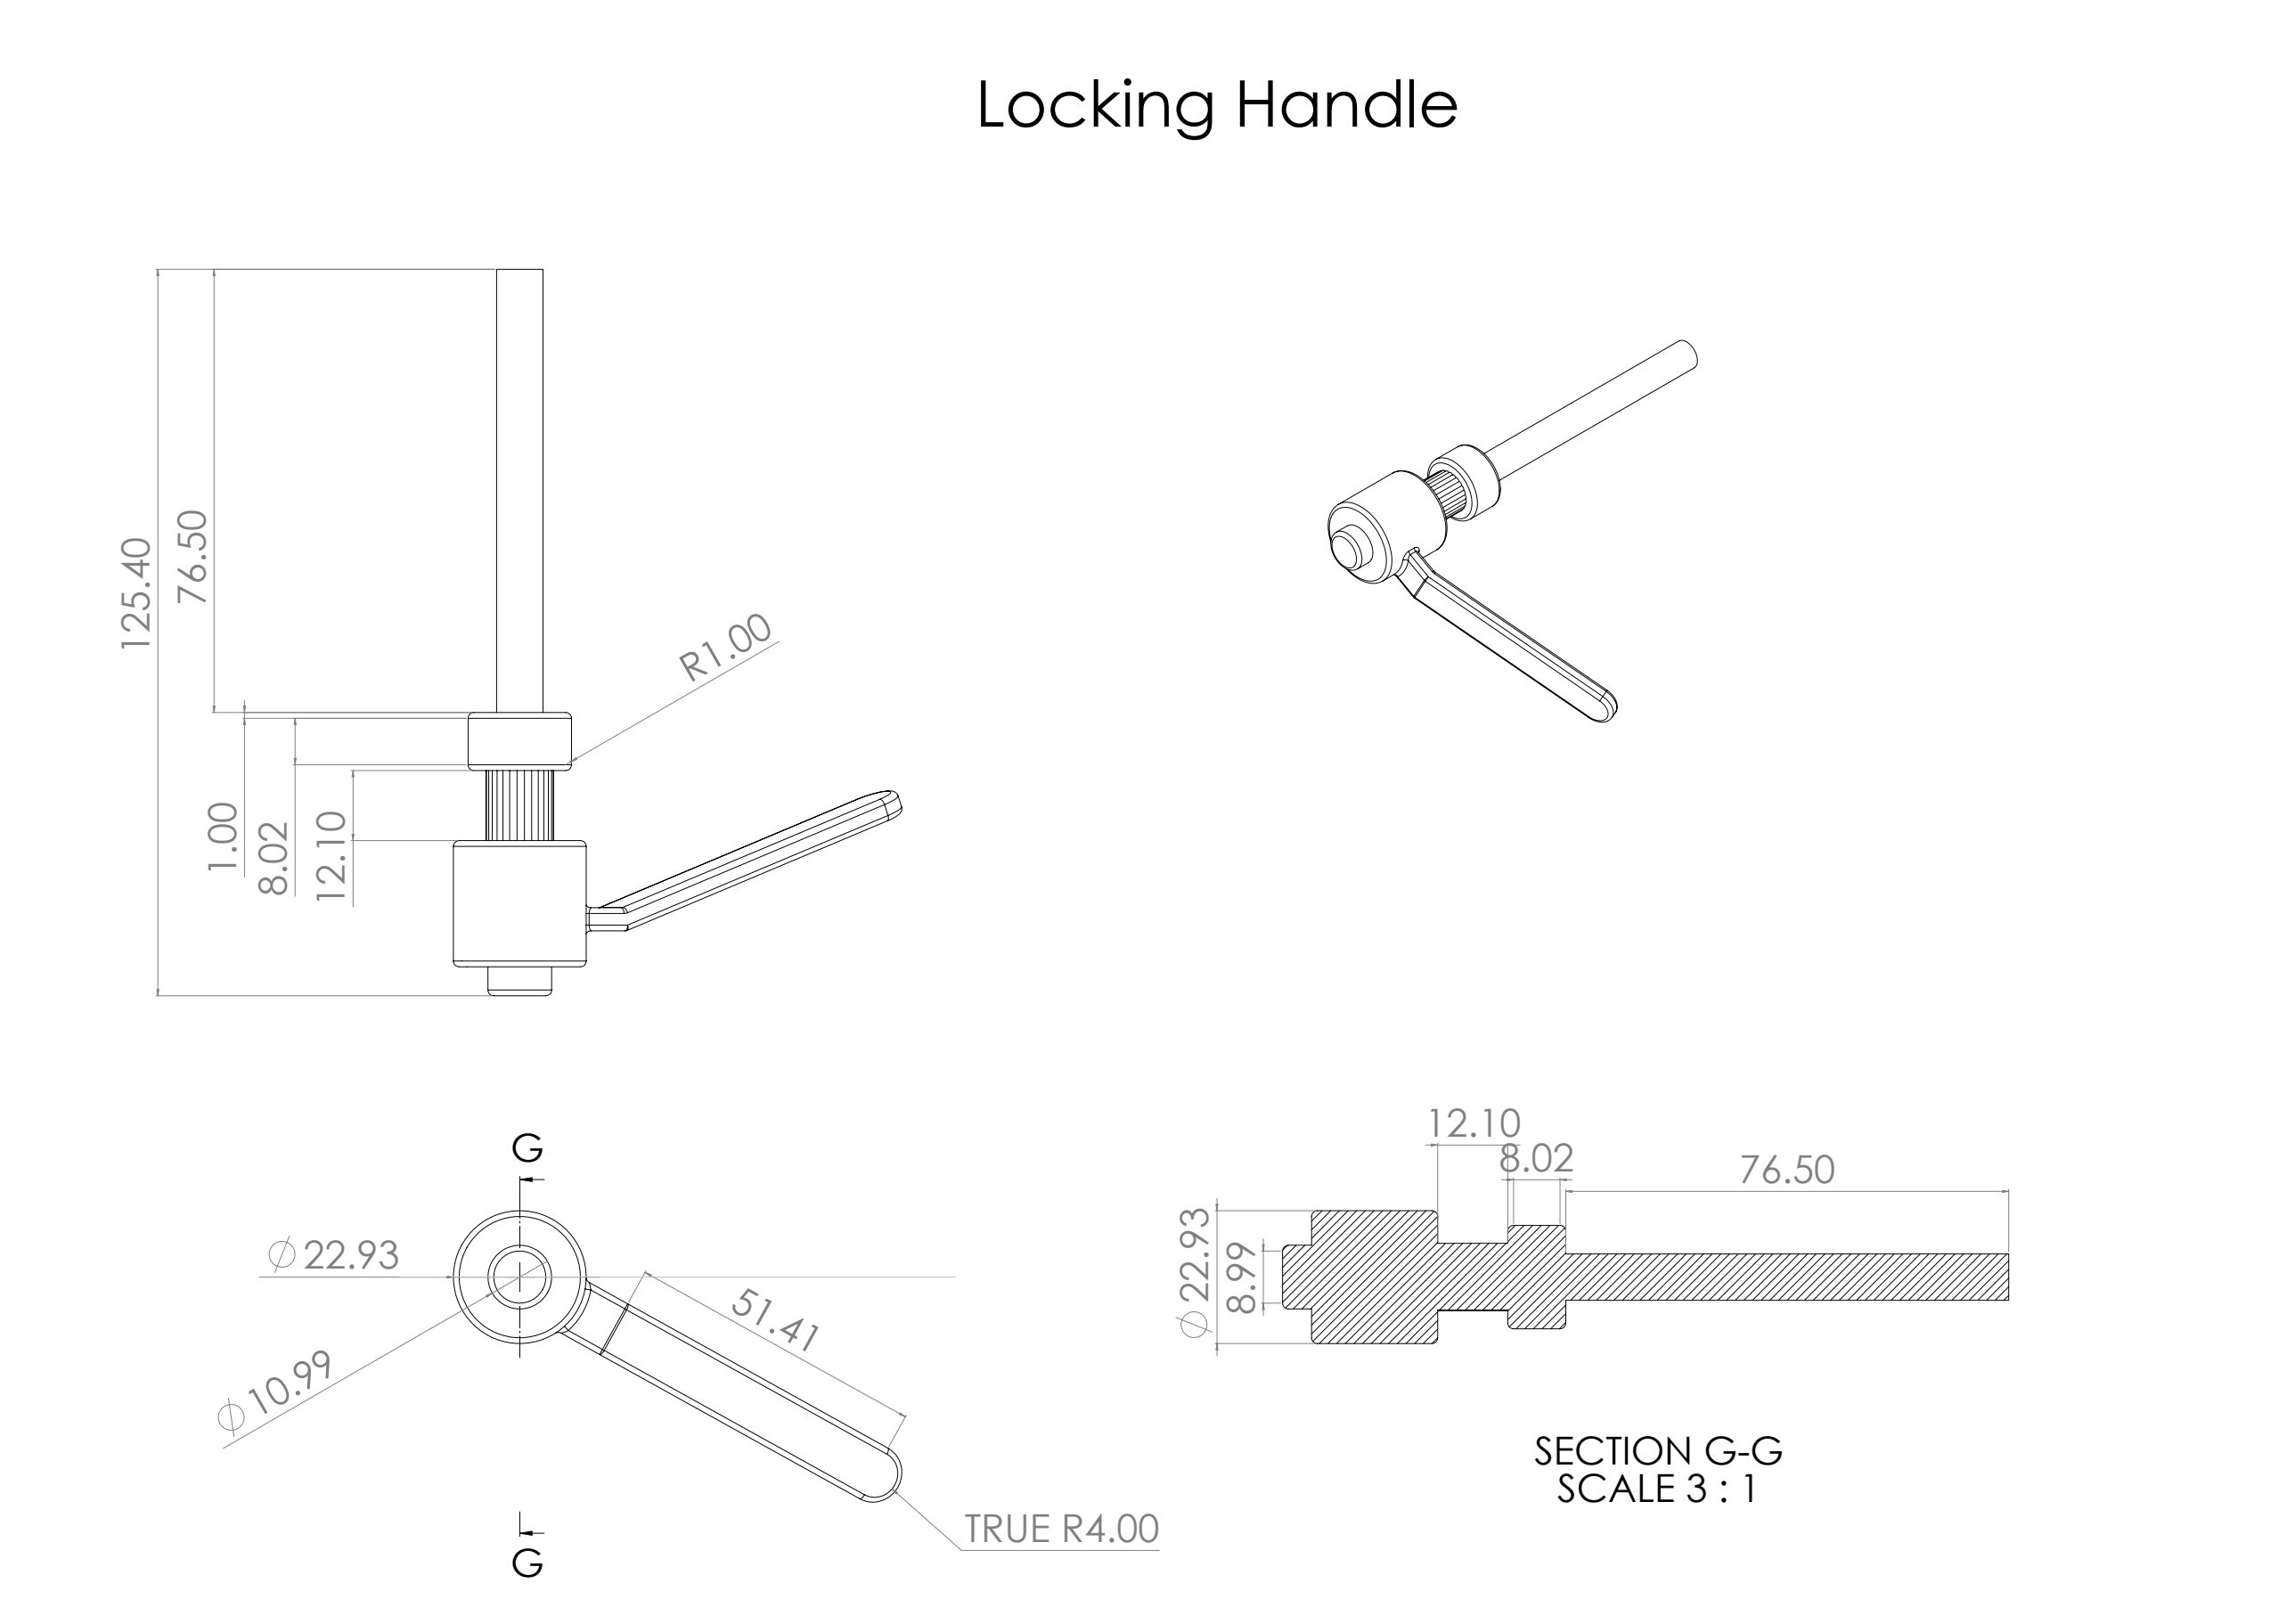
ISO-10303-21;
HEADER;
FILE_DESCRIPTION (('STEP AP214'),
    '1' );
FILE_NAME ('Locking Handle.step',
    '2026-10-24T21:31:31',
    ( '' ),
    ( '' ),
    'SwSTEP 2.0',
    'SolidWorks 2025',
    '' );
FILE_SCHEMA (( 'AUTOMOTIVE_DESIGN' ));
ENDSEC;

DATA;
#2=CARTESIAN_POINT ( 'NONE',  ( 58.00000000000000711, -2.249290599286309256, 86.40005259842790508 ) ) ;
#3=CARTESIAN_POINT ( 'NONE',  ( 58.00000000000000711, -2.249290599286309256, 86.40005259842790508 ) ) ;
#7=CARTESIAN_POINT ( 'NONE',  ( 64.16497654487091040, -11.91588057969686965, 72.65167857827074727 ) ) ;
#22=DIRECTION ( 'NONE',  ( 0.000000000000000000, 0.000000000000000000, -1.000000000000000000 ) ) ;
#23=FACE_OUTER_BOUND ( 'NONE', #14250, .T. ) ;
#26=DIRECTION ( 'NONE',  ( -0.8746197071345572782, 0.4848096202550659650, 1.387778780781444256E-14 ) ) ;
#27=ADVANCED_FACE ( 'NONE', ( #435 ), #1875, .T. ) ;
#30=EDGE_CURVE ( 'NONE', #1762, #13149, #4870, .T. ) ;
#35=CIRCLE ( 'NONE', #11822, 8.924024642120691908 ) ;
#39=DIRECTION ( 'NONE',  ( -0.3020115420618247892, 0.1674077314120183957, -0.9384901064608620613 ) ) ;
#40=CARTESIAN_POINT ( 'NONE',  ( 62.00000000000001421, -2.249290599286311032, -49.31370849898490150 ) ) ;
#43=CARTESIAN_POINT ( 'NONE',  ( 116.3214526938479025, -39.15081599364015119, 53.46824312087640863 ) ) ;
#44=AXIS2_PLACEMENT_3D ( 'NONE', #5649, #10264, #10339 ) ;
#59=VERTEX_POINT ( 'NONE', #10047 ) ;
#61=CARTESIAN_POINT ( 'NONE',  ( 65.61438479068812057, -11.78561916032472823, 75.96106737140233633 ) ) ;
#74=EDGE_CURVE ( 'NONE', #5063, #10163, #11263, .T. ) ;
#76=ORIENTED_EDGE ( 'NONE', *, *, #9899, .T. ) ;
#79=ORIENTED_EDGE ( 'NONE', *, *, #10646, .T. ) ;
#84=DIRECTION ( 'NONE',  ( -0.000000000000000000, 0.000000000000000000, -1.000000000000000000 ) ) ;
#85=ORIENTED_EDGE ( 'NONE', *, *, #4287, .T. ) ;
#100=DIRECTION ( 'NONE',  ( -0.8746197071345569451, 0.4848096202550666312, 0.000000000000000000 ) ) ;
#117=VERTEX_POINT ( 'NONE', #8210 ) ;
#121=CARTESIAN_POINT ( 'NONE',  ( 54.21883389619742388, -5.612936290787406968, 62.84860122826521689 ) ) ;
#124=CARTESIAN_POINT ( 'NONE',  ( 69.30309607900824176, -4.171217477998490075, 76.23845400177138742 ) ) ;
#128=FACE_BOUND ( 'NONE', #8065, .T. ) ;
#136=CARTESIAN_POINT ( 'NONE',  ( 64.12616288941416087, -11.93994285747185913, 75.47114622899779590 ) ) ;
#137=CARTESIAN_POINT ( 'NONE',  ( 65.80512781895316721, -6.575743597179694255, 39.50000000000012790 ) ) ;
#140=ADVANCED_FACE ( 'NONE', ( #6968 ), #10511, .T. ) ;
#141=CARTESIAN_POINT ( 'NONE',  ( 59.31076468612580754, 2.638779099491020297, 60.61639468829817190 ) ) ;
#142=CARTESIAN_POINT ( 'NONE',  ( 67.15257324181105503, -7.322644791425994448, 61.61639468829817190 ) ) ;
#144=CARTESIAN_POINT ( 'NONE',  ( 65.51787304867481510, -10.90583193546819274, 77.18393887567587797 ) ) ;
#147=ORIENTED_EDGE ( 'NONE', *, *, #2886, .F. ) ;
#149=AXIS2_PLACEMENT_3D ( 'NONE', #12314, #13325, #4001 ) ;
#150=ORIENTED_EDGE ( 'NONE', *, *, #12236, .T. ) ;
#152=CARTESIAN_POINT ( 'NONE',  ( 65.93900958890544928, -0.9331851346922672708, 76.19766410831374515 ) ) ;
#153=VERTEX_POINT ( 'NONE', #5752 ) ;
#156=EDGE_LOOP ( 'NONE', ( #7728, #5694, #9406, #597 ) ) ;
#159=TOROIDAL_SURFACE ( 'NONE', #9985, 10.46463184759104870, 1.000000000000000000 ) ;
#178=LINE ( 'NONE', #7254, #6578 ) ;
#179=FACE_OUTER_BOUND ( 'NONE', #4257, .T. ) ;
#185=CARTESIAN_POINT ( 'NONE',  ( 121.8459904851758893, -37.63970102501964021, 53.02550872668530246 ) ) ;
#192=CIRCLE ( 'NONE', #14918, 0.7892041907098250597 ) ;
#195=CARTESIAN_POINT ( 'NONE',  ( 65.61529858912808777, -10.82031860958136704, 71.19766410831375936 ) ) ;
#196=EDGE_CURVE ( 'NONE', #211, #4051, #4578, .T. ) ;
#199=AXIS2_PLACEMENT_3D ( 'NONE', #2893, #5282, #2974 ) ;
#207=EDGE_CURVE ( 'NONE', #5032, #7204, #4344, .T. ) ;
#211=VERTEX_POINT ( 'NONE', #3190 ) ;
#213=DIRECTION ( 'NONE',  ( 0.000000000000000000, 0.000000000000000000, -1.000000000000000000 ) ) ;
#225=ORIENTED_EDGE ( 'NONE', *, *, #12393, .F. ) ;
#230=EDGE_CURVE ( 'NONE', #13103, #13525, #1896, .T. ) ;
#232=DIRECTION ( 'NONE',  ( 0.8746197071345569451, -0.4848096202550666312, 0.000000000000000000 ) ) ;
#233=CARTESIAN_POINT ( 'NONE',  ( 63.00747169918385993, -1.516790343742004055, 62.84860122826521689 ) ) ;
#238=VECTOR ( 'NONE', #7025, 1000.000000000000000 ) ;
#242=EDGE_CURVE ( 'NONE', #604, #9712, #875, .T. ) ;
#243=ORIENTED_EDGE ( 'NONE', *, *, #2367, .F. ) ;
#248=CARTESIAN_POINT ( 'NONE',  ( 53.45023817967523172, -5.433760736713491468, 48.51982618741349285 ) ) ;
#260=AXIS2_PLACEMENT_3D ( 'NONE', #10023, #5325, #2943 ) ;
#268=DIRECTION ( 'NONE',  ( -0.8746197071345569451, 0.4848096202550666312, 0.000000000000000000 ) ) ;
#271=CARTESIAN_POINT ( 'NONE',  ( 69.97972559857380759, -3.172990593254280789, 75.19766410831374515 ) ) ;
#277=ORIENTED_EDGE ( 'NONE', *, *, #11092, .F. ) ;
#279=ORIENTED_EDGE ( 'NONE', *, *, #8747, .F. ) ;
#281=ORIENTED_EDGE ( 'NONE', *, *, #7345, .T. ) ;
#283=CARTESIAN_POINT ( 'NONE',  ( 64.80908095809924419, -11.48972663575131392, 75.86800894915671734 ) ) ;
#285=DIRECTION ( 'NONE',  ( 0.8746197071345571672, -0.4848096202550661871, 0.000000000000000000 ) ) ;
#293=AXIS2_PLACEMENT_3D ( 'NONE', #12680, #6824, #7986 ) ;
#294=DIRECTION ( 'NONE',  ( -0.8746197071345569451, 0.4848096202550666312, 0.000000000000000000 ) ) ;
#297=TOROIDAL_SURFACE ( 'NONE', #10121, 4.496540510819672321, 1.000000000000000000 ) ;
#305=DIRECTION ( 'NONE',  ( 0.000000000000000000, 0.000000000000000000, 1.000000000000000000 ) ) ;
#306=DIRECTION ( 'NONE',  ( -0.000000000000000000, 0.000000000000000000, -1.000000000000000000 ) ) ;
#311=EDGE_CURVE ( 'NONE', #2576, #7654, #192, .T. ) ;
#317=ORIENTED_EDGE ( 'NONE', *, *, #10206, .F. ) ;
#318=VECTOR ( 'NONE', #6465, 1000.000000000000000 ) ;
#327=CYLINDRICAL_SURFACE ( 'NONE', #4362, 1.000000000000005329 ) ;
#334=DIRECTION ( 'NONE',  ( -0.8746197071345570562, 0.4848096202550662981, 0.000000000000000000 ) ) ;
#347=CARTESIAN_POINT ( 'NONE',  ( 69.46221311448613278, -2.886128737383383935, 75.38059407619712715 ) ) ;
#363=DIRECTION ( 'NONE',  ( 0.000000000000000000, 0.000000000000000000, 1.000000000000000000 ) ) ;
#364=EDGE_CURVE ( 'NONE', #14069, #12214, #5110, .T. ) ;
#367=DIRECTION ( 'NONE',  ( 0.000000000000000000, 0.000000000000000000, 1.000000000000000000 ) ) ;
#371=ORIENTED_EDGE ( 'NONE', *, *, #10491, .F. ) ;
#377=DIRECTION ( 'NONE',  ( 0.8746197071345570562, -0.4848096202550665756, 0.000000000000000000 ) ) ;
#381=CYLINDRICAL_SURFACE ( 'NONE', #9577, 11.46463184759105403 ) ;
#382=CARTESIAN_POINT ( 'NONE',  ( 50.19487218104683990, 2.077162398607073968, 82.40005259842790508 ) ) ;
#384=VERTEX_POINT ( 'NONE', #5940 ) ;
#393=DIRECTION ( 'NONE',  ( 1.000000000000000000, 0.000000000000000000, 0.000000000000000000 ) ) ;
#406=CARTESIAN_POINT ( 'NONE',  ( 57.51704887355756313, 3.283153786997079049, 60.61639468829817190 ) ) ;
#408=CYLINDRICAL_SURFACE ( 'NONE', #2891, 1.000000000000000888 ) ;
#412=AXIS2_PLACEMENT_3D ( 'NONE', #11507, #13599, #12438 ) ;
#416=CIRCLE ( 'NONE', #10992, 0.7892041907098262810 ) ;
#421=AXIS2_PLACEMENT_3D ( 'NONE', #800, #5514, #12747 ) ;
#423=VECTOR ( 'NONE', #6451, 1000.000000000000000 ) ;
#435=FACE_OUTER_BOUND ( 'NONE', #6645, .T. ) ;
#437=AXIS2_PLACEMENT_3D ( 'NONE', #3487, #8189, #5565 ) ;
#438=TOROIDAL_SURFACE ( 'NONE', #10274, 12.46463184759105047, 1.000000000000000000 ) ;
#453=LINE ( 'NONE', #3979, #12135 ) ;
#454=EDGE_LOOP ( 'NONE', ( #9894, #4373, #1618, #2467 ) ) ;
#464=DIRECTION ( 'NONE',  ( -0.8208219420614829565, 0.4549890321264266624, 0.3453061251629824246 ) ) ;
#471=EDGE_CURVE ( 'NONE', #12214, #14069, #7553, .T. ) ;
#477=AXIS2_PLACEMENT_3D ( 'NONE', #5498, #9026, #1017 ) ;
#482=DIRECTION ( 'NONE',  ( 1.000000000000000000, 0.000000000000000000, 0.000000000000000000 ) ) ;
#483=CARTESIAN_POINT ( 'NONE',  ( 62.00000000000001421, -2.249290599286311032, -38.00000000000012079 ) ) ;
#489=DIRECTION ( 'NONE',  ( -0.000000000000000000, 0.000000000000000000, -1.000000000000000000 ) ) ;
#496=ORIENTED_EDGE ( 'NONE', *, *, #8220, .F. ) ;
#506=EDGE_LOOP ( 'NONE', ( #7600, #11130, #5855, #5536 ) ) ;
#515=ORIENTED_EDGE ( 'NONE', *, *, #1099, .T. ) ;
#517=DIRECTION ( 'NONE',  ( 0.000000000000000000, 0.000000000000000000, -1.000000000000000000 ) ) ;
#518=EDGE_LOOP ( 'NONE', ( #85, #11509, #6587, #5049 ) ) ;
#524=FACE_BOUND ( 'NONE', #11436, .T. ) ;
#526=CARTESIAN_POINT ( 'NONE',  ( 68.02719294894561131, -7.807454411681060691, 82.40005259842790508 ) ) ;
#536=DIRECTION ( 'NONE',  ( -0.9249888031744268879, 0.3799943604870225089, 0.000000000000000000 ) ) ;
#539=CARTESIAN_POINT ( 'NONE',  ( 64.81656575362153205, -11.48379431191618671, 72.53457481663632223 ) ) ;
#547=CARTESIAN_POINT ( 'NONE',  ( 69.46454297106444642, -2.294433322023684774, 73.19766410831374515 ) ) ;
#553=AXIS2_PLACEMENT_3D ( 'NONE', #1342, #12818, #9352 ) ;
#556=VERTEX_POINT ( 'NONE', #13378 ) ;
#569=ORIENTED_EDGE ( 'NONE', *, *, #14553, .F. ) ;
#597=ORIENTED_EDGE ( 'NONE', *, *, #7672, .F. ) ;
#604=VERTEX_POINT ( 'NONE', #2615 ) ;
#607=DIRECTION ( 'NONE',  ( 0.000000000000000000, 0.000000000000000000, 1.000000000000000000 ) ) ;
#610=ADVANCED_FACE ( 'NONE', ( #2836 ), #381, .T. ) ;
#612=VERTEX_POINT ( 'NONE', #13245 ) ;
#614=CARTESIAN_POINT ( 'NONE',  ( 61.36510378087922390, 1.530577915148011225, 48.51982618741349285 ) ) ;
#629=DIRECTION ( 'NONE',  ( -0.000000000000000000, 0.000000000000000000, -1.000000000000000000 ) ) ;
#635=CARTESIAN_POINT ( 'NONE',  ( 58.00000000000000711, -2.249290599286309256, 61.61639468829817190 ) ) ;
#639=AXIS2_PLACEMENT_3D ( 'NONE', #12293, #305, #1535 ) ;
#644=AXIS2_PLACEMENT_3D ( 'NONE', #12063, #2755, #14382 ) ;
#650=ORIENTED_EDGE ( 'NONE', *, *, #10123, .F. ) ;
#653=EDGE_LOOP ( 'NONE', ( #6707, #7341, #9588, #14019 ) ) ;
#657=CARTESIAN_POINT ( 'NONE',  ( 64.11356537587559501, -11.94785244090458498, 73.19766410831374515 ) ) ;
#667=EDGE_CURVE ( 'NONE', #556, #7206, #3915, .T. ) ;
#679=CARTESIAN_POINT ( 'NONE',  ( 58.00000000000000711, -2.249290599286309256, 39.50000000000012790 ) ) ;
#682=CARTESIAN_POINT ( 'NONE',  ( 54.06723705530823310, -0.06932450177430288241, 87.40005259842790508 ) ) ;
#689=ORIENTED_EDGE ( 'NONE', *, *, #8732, .F. ) ;
#690=CARTESIAN_POINT ( 'NONE',  ( 69.97972559857382180, -3.172990593254281233, 73.19766410831374515 ) ) ;
#691=EDGE_CURVE ( 'NONE', #9315, #7200, #11147, .T. ) ;
#692=ADVANCED_FACE ( 'NONE', ( #8752 ), #5227, .T. ) ;
#695=CARTESIAN_POINT ( 'NONE',  ( 57.83740799265796539, -7.800393779465814248, 48.51982618741349285 ) ) ;
#697=CARTESIAN_POINT ( 'NONE',  ( 55.86211336638498182, 2.337731330496643167, 48.51982618741349285 ) ) ;
#702=DIRECTION ( 'NONE',  ( 0.8746197071345572782, -0.4848096202550659650, 0.000000000000000000 ) ) ;
#706=EDGE_CURVE ( 'NONE', #7249, #2361, #2636, .T. ) ;
#711=CARTESIAN_POINT ( 'NONE',  ( 55.09646579789918519, -6.394265699299607419, 48.51982618741349285 ) ) ;
#713=EDGE_LOOP ( 'NONE', ( #4880, #8165, #76, #1992, #12089, #15118, #2455, #11853, #2027, #8217 ) ) ;
#722=DIRECTION ( 'NONE',  ( -0.8746197071345572782, 0.4848096202550660205, 0.000000000000000000 ) ) ;
#724=CARTESIAN_POINT ( 'NONE',  ( 53.11142512232702018, -3.558169932106523881, 62.84860122826521689 ) ) ;
#739=ORIENTED_EDGE ( 'NONE', *, *, #13013, .T. ) ;
#740=EDGE_CURVE ( 'NONE', #6596, #11588, #12572, .T. ) ;
#742=CARTESIAN_POINT ( 'NONE',  ( 65.13162939602317181, -11.91918766459985157, 75.19766410831374515 ) ) ;
#756=CARTESIAN_POINT ( 'NONE',  ( 52.94134894379979528, -2.395505968190773327, 48.51982618741349285 ) ) ;
#758=AXIS2_PLACEMENT_3D ( 'NONE', #11179, #629, #8952 ) ;
#760=AXIS2_PLACEMENT_3D ( 'NONE', #3547, #3770, #5009 ) ;
#761=ORIENTED_EDGE ( 'NONE', *, *, #10485, .F. ) ;
#762=CARTESIAN_POINT ( 'NONE',  ( 69.99788034154117611, -3.225610097367463514, 75.50178636978743896 ) ) ;
#772=ORIENTED_EDGE ( 'NONE', *, *, #1941, .T. ) ;
#775=CARTESIAN_POINT ( 'NONE',  ( 52.25109540565180311, -2.012892184189035039, 62.84860122826521689 ) ) ;
#786=CYLINDRICAL_SURFACE ( 'NONE', #758, 0.7892041907098262810 ) ;
#787=ORIENTED_EDGE ( 'NONE', *, *, #10191, .T. ) ;
#795=CARTESIAN_POINT ( 'NONE',  ( 56.97758043373130477, 2.707118148285912795, 60.61639468829817190 ) ) ;
#796=DIRECTION ( 'NONE',  ( -0.000000000000000000, 0.000000000000000000, -1.000000000000000000 ) ) ;
#800=CARTESIAN_POINT ( 'NONE',  ( 62.80358567007132820, -3.842053655357405173, 60.61639468829817190 ) ) ;
#807=ORIENTED_EDGE ( 'NONE', *, *, #6638, .F. ) ;
#818=VECTOR ( 'NONE', #7680, 1000.000000000000000 ) ;
#819=FACE_OUTER_BOUND ( 'NONE', #7730, .T. ) ;
#833=CARTESIAN_POINT ( 'NONE',  ( 121.4079758241357609, -32.82348926221179397, 57.22220354671984666 ) ) ;
#846=CARTESIAN_POINT ( 'NONE',  ( 69.45807991563580686, -2.948854807202607731, 72.84297311730249191 ) ) ;
#852=ORIENTED_EDGE ( 'NONE', *, *, #5942, .T. ) ;
#854=( LENGTH_UNIT ( ) NAMED_UNIT ( * ) SI_UNIT ( .MILLI., .METRE. ) );
#858=ORIENTED_EDGE ( 'NONE', *, *, #14035, .T. ) ;
#860=DIRECTION ( 'NONE',  ( 0.9839406800755990945, -0.1784957649143745217, 0.000000000000000000 ) ) ;
#861=DIRECTION ( 'NONE',  ( -0.000000000000000000, 0.000000000000000000, -1.000000000000000000 ) ) ;
#865=ORIENTED_EDGE ( 'NONE', *, *, #8044, .F. ) ;
#873=CARTESIAN_POINT ( 'NONE',  ( 116.1386546156546444, -40.19284343218672007, 54.40673322733725570 ) ) ;
#875=LINE ( 'NONE', #15126, #9021 ) ;
#879=VERTEX_POINT ( 'NONE', #7688 ) ;
#885=CIRCLE ( 'NONE', #12695, 0.7892041907098275022 ) ;
#889=DIRECTION ( 'NONE',  ( 0.000000000000000000, 0.000000000000000000, 1.000000000000000000 ) ) ;
#899=FACE_OUTER_BOUND ( 'NONE', #4695, .T. ) ;
#900=ORIENTED_EDGE ( 'NONE', *, *, #4035, .F. ) ;
#909=AXIS2_PLACEMENT_3D ( 'NONE', #991, #9316, #8085 ) ;
#910=VECTOR ( 'NONE', #6269, 999.9999999999998863 ) ;
#924=CARTESIAN_POINT ( 'NONE',  ( 69.28051765693513175, -4.295678830383772961, 72.19766410831373094 ) ) ;
#931=VERTEX_POINT ( 'NONE', #8912 ) ;
#932=VECTOR ( 'NONE', #5247, 1000.000000000000000 ) ;
#940=ORIENTED_EDGE ( 'NONE', *, *, #12365, .F. ) ;
#943=VERTEX_POINT ( 'NONE', #12611 ) ;
#947=CARTESIAN_POINT ( 'NONE',  ( 60.05137561479872232, 2.911430354694811484, 48.51982618741349285 ) ) ;
#948=DIRECTION ( 'NONE',  ( -0.000000000000000000, 0.000000000000000000, -1.000000000000000000 ) ) ;
#959=ORIENTED_EDGE ( 'NONE', *, *, #13649, .F. ) ;
#978=DIRECTION ( 'NONE',  ( 0.3020115420618247892, -0.1674077314120183957, 0.9384901064608620613 ) ) ;
#983=DIRECTION ( 'NONE',  ( -0.4848096202550659650, -0.8746197071345572782, 0.000000000000000000 ) ) ;
#985=CARTESIAN_POINT ( 'NONE',  ( 54.00000000000000711, -2.249290599286310588, -49.31370849898490150 ) ) ;
#991=CARTESIAN_POINT ( 'NONE',  ( 58.00000000000000711, -2.249290599286311032, 38.50000000000012790 ) ) ;
#993=CARTESIAN_POINT ( 'NONE',  ( 69.41637355099324225, -3.305665566658139376, 76.92699484961572409 ) ) ;
#996=VERTEX_POINT ( 'NONE', #9154 ) ;
#999=AXIS2_PLACEMENT_3D ( 'NONE', #14231, #1449, #6157 ) ;
#1005=AXIS2_PLACEMENT_3D ( 'NONE', #15165, #10318, #12789 ) ;
#1010=EDGE_CURVE ( 'NONE', #879, #9712, #9431, .T. ) ;
#1016=CIRCLE ( 'NONE', #2502, 5.496540510819668768 ) ;
#1017=DIRECTION ( 'NONE',  ( 0.3020115420618323387, -0.1674077314120217264, 0.9384901064608589527 ) ) ;
#1020=ORIENTED_EDGE ( 'NONE', *, *, #14571, .F. ) ;
#1023=ORIENTED_EDGE ( 'NONE', *, *, #15171, .T. ) ;
#1024=DIRECTION ( 'NONE',  ( 0.1784957649143733838, 0.9839406800755994276, -0.000000000000000000 ) ) ;
#1033=DIRECTION ( 'NONE',  ( 0.8746197071345573892, -0.4848096202550657430, 0.000000000000000000 ) ) ;
#1040=EDGE_CURVE ( 'NONE', #12282, #6181, #9065, .T. ) ;
#1043=EDGE_CURVE ( 'NONE', #604, #5327, #4004, .T. ) ;
#1051=CARTESIAN_POINT ( 'NONE',  ( 68.02719294894561131, -7.807454411681058026, 81.40005259842790508 ) ) ;
#1052=DIRECTION ( 'NONE',  ( 0.000000000000000000, 0.000000000000000000, 1.000000000000000000 ) ) ;
#1056=ORIENTED_EDGE ( 'NONE', *, *, #10977, .T. ) ;
#1064=ORIENTED_EDGE ( 'NONE', *, *, #11189, .T. ) ;
#1065=DIRECTION ( 'NONE',  ( 0.000000000000000000, 0.000000000000000000, 1.000000000000000000 ) ) ;
#1067=CIRCLE ( 'NONE', #10913, 0.7892041907098261699 ) ;
#1068=EDGE_CURVE ( 'NONE', #2182, #12939, #10900, .T. ) ;
#1072=DIRECTION ( 'NONE',  ( -0.000000000000000000, 0.000000000000000000, -1.000000000000000000 ) ) ;
#1073=LINE ( 'NONE', #10467, #9643 ) ;
#1075=ORIENTED_EDGE ( 'NONE', *, *, #10722, .F. ) ;
#1077=CARTESIAN_POINT ( 'NONE',  ( 64.65840159946851884, -11.60091655178341696, 72.83455400280563197 ) ) ;
#1078=DIRECTION ( 'NONE',  ( 0.3020115420618247892, -0.1674077314120183957, 0.9384901064608620613 ) ) ;
#1087=DIRECTION ( 'NONE',  ( 0.000000000000000000, 0.000000000000000000, 1.000000000000000000 ) ) ;
#1088=CARTESIAN_POINT ( 'NONE',  ( 56.56161818778031858, -7.613266777470379942, 54.56811043785582882 ) ) ;
#1093=CARTESIAN_POINT ( 'NONE',  ( 54.30726695196912601, -6.397170215889376621, 60.61639468829817190 ) ) ;
#1094=CARTESIAN_POINT ( 'NONE',  ( 52.72873328492558187, -0.5014548242779776066, 54.56811043785582882 ) ) ;
#1099=EDGE_CURVE ( 'NONE', #3217, #9619, #12876, .T. ) ;
#1103=ORIENTED_EDGE ( 'NONE', *, *, #3765, .F. ) ;
#1118=FACE_OUTER_BOUND ( 'NONE', #3433, .T. ) ;
#1119=EDGE_CURVE ( 'NONE', #1157, #384, #4495, .T. ) ;
#1123=EDGE_CURVE ( 'NONE', #5327, #943, #11624, .T. ) ;
#1126=DIRECTION ( 'NONE',  ( 0.000000000000000000, 0.000000000000000000, 1.000000000000000000 ) ) ;
#1128=DIRECTION ( 'NONE',  ( 0.8746197071345569451, -0.4848096202550666312, 0.000000000000000000 ) ) ;
#1129=CYLINDRICAL_SURFACE ( 'NONE', #6973, 1.000000000000000444 ) ;
#1136=PLANE ( 'NONE',  #5436 ) ;
#1138=EDGE_LOOP ( 'NONE', ( #6793, #4822, #4988, #10304 ) ) ;
#1140=CARTESIAN_POINT ( 'NONE',  ( 54.17164678268019173, 2.103670757168142114, 60.61639468829817190 ) ) ;
#1147=AXIS2_PLACEMENT_3D ( 'NONE', #7440, #3671, #285 ) ;
#1154=DIRECTION ( 'NONE',  ( -0.8746197071345569451, 0.4848096202550666312, 0.000000000000000000 ) ) ;
#1157=VERTEX_POINT ( 'NONE', #6907 ) ;
#1168=ORIENTED_EDGE ( 'NONE', *, *, #11677, .T. ) ;
#1179=DIRECTION ( 'NONE',  ( -0.000000000000000000, 0.000000000000000000, -1.000000000000000000 ) ) ;
#1185=DIRECTION ( 'NONE',  ( -0.000000000000000000, -0.000000000000000000, -1.000000000000000000 ) ) ;
#1191=CARTESIAN_POINT ( 'NONE',  ( 71.15942379059755751, -15.26044865788734484, 71.19766410831374515 ) ) ;
#1192=DIRECTION ( 'NONE',  ( 0.000000000000000000, 0.000000000000000000, 1.000000000000000000 ) ) ;
#1207=CARTESIAN_POINT ( 'NONE',  ( 65.18141112804345028, -11.90723896596971798, 75.46703592544538708 ) ) ;
#1213=AXIS2_PLACEMENT_3D ( 'NONE', #5888, #13034, #4946 ) ;
#1214=CIRCLE ( 'NONE', #477, 0.9999999999999948930 ) ;
#1217=CARTESIAN_POINT ( 'NONE',  ( 65.32299310458444097, -11.07130256205453200, 77.13099622499589714 ) ) ;
#1219=CARTESIAN_POINT ( 'NONE',  ( 4.848008884920353090, 21.49656883983473676, 0.000000000000000000 ) ) ;
#1227=TOROIDAL_SURFACE ( 'NONE', #6624, 10.46463184759104870, 1.000000000000000000 ) ;
#1229=CARTESIAN_POINT ( 'NONE',  ( 69.97972559857382180, -3.172990593254279457, 73.19766410831374515 ) ) ;
#1230=ORIENTED_EDGE ( 'NONE', *, *, #9692, .T. ) ;
#1232=LINE ( 'NONE', #382, #3479 ) ;
#1233=CARTESIAN_POINT ( 'NONE',  ( 47.97280705105441001, 3.308873213108444400, 61.61639468829817190 ) ) ;
#1235=CARTESIAN_POINT ( 'NONE',  ( 69.41342053903602505, -3.337090261597983609, 71.45041864562929845 ) ) ;
#1240=DIRECTION ( 'NONE',  ( 0.8746197071345569451, -0.4848096202550666312, 0.000000000000000000 ) ) ;
#1243=CARTESIAN_POINT ( 'NONE',  ( 61.57572300660984865, -8.804762498903286883, 75.19766410831374515 ) ) ;
#1255=DIRECTION ( 'NONE',  ( -0.8746197071345555019, 0.4848096202550691847, 0.000000000000000000 ) ) ;
#1260=LINE ( 'NONE', #5974, #11225 ) ;
#1266=AXIS2_PLACEMENT_3D ( 'NONE', #2022, #489, #12411 ) ;
#1267=DIRECTION ( 'NONE',  ( 0.8746197071345570562, -0.4848096202550665756, 0.000000000000000000 ) ) ;
#1269=PLANE ( 'NONE',  #7327 ) ;
#1281=CARTESIAN_POINT ( 'NONE',  ( 72.42321995572909543, -14.81762824354790276, 76.19766410831374515 ) ) ;
#1284=VECTOR ( 'NONE', #12777, 1000.000000000000000 ) ;
#1287=DIRECTION ( 'NONE',  ( 0.8746197071345572782, -0.4848096202550659650, 0.000000000000000000 ) ) ;
#1290=EDGE_LOOP ( 'NONE', ( #3521, #15102, #569, #10478, #1685 ) ) ;
#1293=DIRECTION ( 'NONE',  ( 0.000000000000000000, 0.000000000000000000, 1.000000000000000000 ) ) ;
#1294=ORIENTED_EDGE ( 'NONE', *, *, #2324, .T. ) ;
#1298=ORIENTED_EDGE ( 'NONE', *, *, #8807, .T. ) ;
#1301=FACE_OUTER_BOUND ( 'NONE', #10786, .T. ) ;
#1303=VECTOR ( 'NONE', #9531, 1000.000000000000000 ) ;
#1306=ORIENTED_EDGE ( 'NONE', *, *, #10977, .F. ) ;
#1313=CARTESIAN_POINT ( 'NONE',  ( 65.13162939602315760, -11.91918766459984980, 73.04333912804901274 ) ) ;
#1314=AXIS2_PLACEMENT_3D ( 'NONE', #6602, #11288, #7612 ) ;
#1319=SHAPE_REPRESENTATION_RELATIONSHIP ( 'NONE' , 'NONE' ,  #11972, #8677 ) ;
#1321=EDGE_CURVE ( 'NONE', #7274, #6176, #11638, .T. ) ;
#1322=CARTESIAN_POINT ( 'NONE',  ( 121.1059642820739128, -32.65608153079976006, 56.28371344025897827 ) ) ;
#1336=ORIENTED_EDGE ( 'NONE', *, *, #11677, .F. ) ;
#1338=ORIENTED_EDGE ( 'NONE', *, *, #1702, .T. ) ;
#1342=CARTESIAN_POINT ( 'NONE',  ( 60.65595175199513278, -6.557103238384438981, 62.84860122826521689 ) ) ;
#1344=CARTESIAN_POINT ( 'NONE',  ( 70.18595114983344274, -3.932849470457435714, 76.10019179193449190 ) ) ;
#1348=DIRECTION ( 'NONE',  ( -0.000000000000000000, 0.000000000000000000, -1.000000000000000000 ) ) ;
#1358=CARTESIAN_POINT ( 'NONE',  ( 65.71319926014257362, -10.73129157630436659, 77.19766410831375936 ) ) ;
#1370=EDGE_LOOP ( 'NONE', ( #3463, #12064, #11267, #9958 ) ) ;
#1374=AXIS2_PLACEMENT_3D ( 'NONE', #6468, #8766, #7549 ) ;
#1380=CARTESIAN_POINT ( 'NONE',  ( 59.31076468612580754, 2.638779099491020297, 48.51982618741349285 ) ) ;
#1404=DIRECTION ( 'NONE',  ( 0.8746197071345563900, -0.4848096202550675193, 0.000000000000000000 ) ) ;
#1406=CIRCLE ( 'NONE', #12459, 4.999999999999997335 ) ;
#1408=CARTESIAN_POINT ( 'NONE',  ( 69.46454297106444642, -2.294433322023680333, 82.40005259842790508 ) ) ;
#1416=CIRCLE ( 'NONE', #14450, 12.46463184759105047 ) ;
#1419=EDGE_CURVE ( 'NONE', #3763, #13687, #1067, .T. ) ;
#1420=CARTESIAN_POINT ( 'NONE',  ( 65.61961478802662384, -10.81639363244362428, 72.15687421485361597 ) ) ;
#1423=AXIS2_PLACEMENT_3D ( 'NONE', #6574, #5131, #1812 ) ;
#1425=AXIS2_PLACEMENT_3D ( 'NONE', #6810, #4505, #5756 ) ;
#1427=DIRECTION ( 'NONE',  ( 0.000000000000000000, 0.000000000000000000, -1.000000000000000000 ) ) ;
#1436=FACE_OUTER_BOUND ( 'NONE', #5190, .T. ) ;
#1439=CIRCLE ( 'NONE', #5620, 1.000000000000001998 ) ;
#1447=CARTESIAN_POINT ( 'NONE',  ( 65.71319926014255941, -10.73129157630437547, 77.19766410831374515 ) ) ;
#1449=DIRECTION ( 'NONE',  ( -0.000000000000000000, 0.000000000000000000, -1.000000000000000000 ) ) ;
#1459=DIRECTION ( 'NONE',  ( 0.8746197071345569451, -0.4848096202550666312, 0.000000000000000000 ) ) ;
#1461=ADVANCED_FACE ( 'NONE', ( #5517 ), #4343, .T. ) ;
#1470=DIRECTION ( 'NONE',  ( -0.8208219420614785156, 0.4549890321264269399, 0.3453061251629920836 ) ) ;
#1478=CARTESIAN_POINT ( 'NONE',  ( 63.03271294676726910, -4.597264848142483373, 60.61639468829817190 ) ) ;
#1483=CYLINDRICAL_SURFACE ( 'NONE', #13489, 5.496540510819668768 ) ;
#1496=CARTESIAN_POINT ( 'NONE',  ( 69.44353280118474459, -3.136524796243262525, 75.86075339999212019 ) ) ;
#1498=CARTESIAN_POINT ( 'NONE',  ( 64.55850009422569258, -11.65316488165094100, 71.85201186900997072 ) ) ;
#1500=CARTESIAN_POINT ( 'NONE',  ( 55.86211336638498182, 2.337731330496643167, 48.51982618741349285 ) ) ;
#1502=CARTESIAN_POINT ( 'NONE',  ( 69.45547845231760675, -2.986442851882156191, 72.75847651673318239 ) ) ;
#1504=DIRECTION ( 'NONE',  ( -1.000000000000000000, 0.000000000000000000, 0.000000000000000000 ) ) ;
#1523=CYLINDRICAL_SURFACE ( 'NONE', #3638, 0.7892041907098262810 ) ;
#1525=ORIENTED_EDGE ( 'NONE', *, *, #2199, .T. ) ;
#1526=CARTESIAN_POINT ( 'NONE',  ( 64.11356537587556659, -11.94785244090457965, 75.32972112861136793 ) ) ;
#1528=EDGE_LOOP ( 'NONE', ( #1020, #1525, #5297, #14230 ) ) ;
#1530=LINE ( 'NONE', #1675, #8433 ) ;
#1534=AXIS2_PLACEMENT_3D ( 'NONE', #5720, #3320, #6855 ) ;
#1535=DIRECTION ( 'NONE',  ( 0.8746197071345569451, -0.4848096202550666312, 0.000000000000000000 ) ) ;
#1545=EDGE_LOOP ( 'NONE', ( #14504, #787, #1294, #11197 ) ) ;
#1546=AXIS2_PLACEMENT_3D ( 'NONE', #1693, #10005, #10080 ) ;
#1547=DIRECTION ( 'NONE',  ( -1.000000000000000000, 0.000000000000000000, 0.000000000000000000 ) ) ;
#1563=AXIS2_PLACEMENT_3D ( 'NONE', #4624, #8170, #11384 ) ;
#1574=CARTESIAN_POINT ( 'NONE',  ( 69.44830357739648719, -3.079170558718888007, 75.78944312221568680 ) ) ;
#1577=FACE_OUTER_BOUND ( 'NONE', #10763, .T. ) ;
#1582=VERTEX_POINT ( 'NONE', #3277 ) ;
#1585=VERTEX_POINT ( 'NONE', #7975 ) ;
#1587=VERTEX_POINT ( 'NONE', #4661 ) ;
#1590=ORIENTED_EDGE ( 'NONE', *, *, #13873, .F. ) ;
#1594=ORIENTED_EDGE ( 'NONE', *, *, #4562, .T. ) ;
#1595=ORIENTED_EDGE ( 'NONE', *, *, #14496, .F. ) ;
#1599=FACE_OUTER_BOUND ( 'NONE', #1545, .T. ) ;
#1600=VERTEX_POINT ( 'NONE', #15053 ) ;
#1601=DIRECTION ( 'NONE',  ( 0.9816271834495682302, 0.1908089953667485572, 0.000000000000000000 ) ) ;
#1603=EDGE_CURVE ( 'NONE', #13714, #11917, #14688, .T. ) ;
#1610=ADVANCED_FACE ( 'NONE', ( #5982, #128 ), #1269, .F. ) ;
#1617=ORIENTED_EDGE ( 'NONE', *, *, #311, .T. ) ;
#1618=ORIENTED_EDGE ( 'NONE', *, *, #5942, .F. ) ;
#1623=FACE_OUTER_BOUND ( 'NONE', #5230, .T. ) ;
#1633=CIRCLE ( 'NONE', #11945, 0.7892041907098272802 ) ;
#1635=ORIENTED_EDGE ( 'NONE', *, *, #471, .T. ) ;
#1639=CARTESIAN_POINT ( 'NONE',  ( 54.06723705530823310, -0.06932450177430304894, 86.40005259842790508 ) ) ;
#1642=CARTESIAN_POINT ( 'NONE',  ( 64.11356537587560922, -11.94785244090458498, 73.06537742987060824 ) ) ;
#1649=ORIENTED_EDGE ( 'NONE', *, *, #8333, .T. ) ;
#1656=EDGE_CURVE ( 'NONE', #12140, #10521, #13236, .T. ) ;
#1657=AXIS2_PLACEMENT_3D ( 'NONE', #14633, #10959, #8784 ) ;
#1659=LINE ( 'NONE', #6354, #12590 ) ;
#1664=VECTOR ( 'NONE', #4909, 1000.000000000000000 ) ;
#1675=CARTESIAN_POINT ( 'NONE',  ( 120.1999296558884254, -32.15385833656369385, 53.46824312087640863 ) ) ;
#1680=CIRCLE ( 'NONE', #6838, 7.924024642120691908 ) ;
#1685=ORIENTED_EDGE ( 'NONE', *, *, #6230, .F. ) ;
#1693=CARTESIAN_POINT ( 'NONE',  ( 58.00000000000000711, -2.249290599286309256, 60.61639468829817190 ) ) ;
#1695=CARTESIAN_POINT ( 'NONE',  ( 37.90194648202322014, 13.46465865409118834, 89.15517579724127017 ) ) ;
#1701=CARTESIAN_POINT ( 'NONE',  ( 49.07597535787931520, -2.249290599286308368, 39.50000000000012790 ) ) ;
#1702=EDGE_CURVE ( 'NONE', #3976, #2824, #2890, .T. ) ;
#1711=DIRECTION ( 'NONE',  ( 0.4848096202550661871, 0.8746197071345573892, -0.000000000000000000 ) ) ;
#1746=CARTESIAN_POINT ( 'NONE',  ( 69.30409605188944511, -4.165705203404209023, 71.19766410831373094 ) ) ;
#1751=VECTOR ( 'NONE', #2028, 1000.000000000000000 ) ;
#1756=DIRECTION ( 'NONE',  ( 0.000000000000000000, 0.000000000000000000, 1.000000000000000000 ) ) ;
#1759=EDGE_CURVE ( 'NONE', #12282, #6287, #1910, .T. ) ;
#1762=VERTEX_POINT ( 'NONE', #4318 ) ;
#1765=CARTESIAN_POINT ( 'NONE',  ( 54.17164678268019173, 2.103670757168141670, 62.84860122826521689 ) ) ;
#1768=CARTESIAN_POINT ( 'NONE',  ( 69.97972559857382180, -3.172990593254279457, 0.000000000000000000 ) ) ;
#1774=FACE_OUTER_BOUND ( 'NONE', #5288, .T. ) ;
#1775=TOROIDAL_SURFACE ( 'NONE', #9866, 4.496540510819672321, 1.000000000000000000 ) ;
#1778=CIRCLE ( 'NONE', #4219, 12.46463184759105047 ) ;
#1782=CARTESIAN_POINT ( 'NONE',  ( 55.17185982823698964, 2.720345114498381456, 60.61639468829817190 ) ) ;
#1783=ADVANCED_FACE ( 'NONE', ( #10260 ), #14952, .T. ) ;
#1786=AXIS2_PLACEMENT_3D ( 'NONE', #3044, #13732, #13805 ) ;
#1787=DIRECTION ( 'NONE',  ( 0.000000000000000000, 0.000000000000000000, 1.000000000000000000 ) ) ;
#1792=EDGE_CURVE ( 'NONE', #7274, #7793, #4055, .T. ) ;
#1795=FACE_OUTER_BOUND ( 'NONE', #4569, .T. ) ;
#1812=DIRECTION ( 'NONE',  ( 0.000000000000000000, -5.204170427930416550E-15, -1.000000000000000000 ) ) ;
#1815=FACE_OUTER_BOUND ( 'NONE', #9374, .T. ) ;
#1818=ORIENTED_EDGE ( 'NONE', *, *, #10407, .T. ) ;
#1824=CARTESIAN_POINT ( 'NONE',  ( 69.46454297106444642, -2.294433322023680333, 75.19766410831374515 ) ) ;
#1829=EDGE_CURVE ( 'NONE', #5327, #2379, #178, .T. ) ;
#1836=ORIENTED_EDGE ( 'NONE', *, *, #5241, .F. ) ;
#1849=CARTESIAN_POINT ( 'NONE',  ( 61.44362764059101067, -6.606194471396438672, 48.51982618741349285 ) ) ;
#1855=CARTESIAN_POINT ( 'NONE',  ( 121.5907739023289906, -31.78146182366520378, 56.28371344025897827 ) ) ;
#1867=DIRECTION ( 'NONE',  ( -0.000000000000000000, 0.000000000000000000, -1.000000000000000000 ) ) ;
#1875=CYLINDRICAL_SURFACE ( 'NONE', #8063, 0.7892041907098262810 ) ;
#1876=DIRECTION ( 'NONE',  ( 0.000000000000000000, 0.000000000000000000, -1.000000000000000000 ) ) ;
#1881=EDGE_CURVE ( 'NONE', #8779, #9351, #4679, .T. ) ;
#1882=ORIENTED_EDGE ( 'NONE', *, *, #5241, .T. ) ;
#1884=AXIS2_PLACEMENT_3D ( 'NONE', #7493, #14711, #482 ) ;
#1886=VERTEX_POINT ( 'NONE', #6651 ) ;
#1889=CARTESIAN_POINT ( 'NONE',  ( 54.30726695196912601, -6.397170215889376621, 54.56811043785582882 ) ) ;
#1896=CIRCLE ( 'NONE', #6811, 8.924024642120691908 ) ;
#1900=CARTESIAN_POINT ( 'NONE',  ( 62.88869237673507229, 0.3854521819929429549, 60.61639468829817190 ) ) ;
#1901=CARTESIAN_POINT ( 'NONE',  ( 53.41380296247595538, -0.1096349785133995947, 62.84860122826521689 ) ) ;
#1902=DIRECTION ( 'NONE',  ( -0.01745240642731254316, 0.9998476951565652415, 0.000000000000000000 ) ) ;
#1903=CARTESIAN_POINT ( 'NONE',  ( 58.00000000000000711, -2.249290599286311032, -38.00000000000012079 ) ) ;
#1910=CIRCLE ( 'NONE', #437, 11.46463184759105403 ) ;
#1925=CARTESIAN_POINT ( 'NONE',  ( 69.46406466716308614, -2.366909661580891999, 72.65892047407166388 ) ) ;
#1933=CYLINDRICAL_SURFACE ( 'NONE', #12594, 0.7892041907098262810 ) ;
#1941=EDGE_CURVE ( 'NONE', #384, #14607, #5874, .T. ) ;
#1946=ORIENTED_EDGE ( 'NONE', *, *, #207, .F. ) ;
#1950=AXIS2_PLACEMENT_3D ( 'NONE', #3567, #15192, #2641 ) ;
#1971=ADVANCED_FACE ( 'NONE', ( #10048 ), #12232, .T. ) ;
#1984=ORIENTED_EDGE ( 'NONE', *, *, #471, .F. ) ;
#1990=CIRCLE ( 'NONE', #12570, 0.7892041907098262810 ) ;
#1991=CARTESIAN_POINT ( 'NONE',  ( 53.41380296247595538, -0.1096349785133995947, 60.61639468829817190 ) ) ;
#1992=ORIENTED_EDGE ( 'NONE', *, *, #6390, .F. ) ;
#1998=VERTEX_POINT ( 'NONE', #6049 ) ;
#2008=DIRECTION ( 'NONE',  ( 0.000000000000000000, 0.000000000000000000, 1.000000000000000000 ) ) ;
#2011=DIRECTION ( 'NONE',  ( 0.4848096202550659650, 0.8746197071345572782, -0.000000000000000000 ) ) ;
#2014=AXIS2_PLACEMENT_3D ( 'NONE', #10154, #15082, #14841 ) ;
#2016=EDGE_CURVE ( 'NONE', #8583, #13229, #9550, .T. ) ;
#2022=CARTESIAN_POINT ( 'NONE',  ( 62.80358567007132820, -3.842053655357405173, 62.84860122826521689 ) ) ;
#2027=ORIENTED_EDGE ( 'NONE', *, *, #10558, .T. ) ;
#2028=DIRECTION ( 'NONE',  ( 0.8746197071345572782, -0.4848096202550659650, -0.000000000000000000 ) ) ;
#2035=( BOUNDED_SURFACE ( )  B_SPLINE_SURFACE ( 3, 2, ( 
 ( #4434, #9142, #13828 ),
 ( #14358, #124, #8357 ),
 ( #12029, #3800, #7266 ),
 ( #2427, #2579, #1344 ),
 ( #8504, #8435, #4808 ),
 ( #13125, #10891, #7118 ),
 ( #12976, #4888, #13047 ),
 ( #8571, #9507, #10663 ),
 ( #9437, #12115, #13194 ),
 ( #3875, #1496, #13270 ),
 ( #11804, #1574, #2719 ),
 ( #6203, #7420, #11954 ),
 ( #2653, #347, #5037 ),
 ( #6270, #7342, #271 ) ),
 .UNSPECIFIED., .F., .F., .F. ) 
 B_SPLINE_SURFACE_WITH_KNOTS ( ( 4, 2, 2, 2, 2, 2, 4 ),
 ( 3, 3 ),
 ( 0.001417163504557061859, 0.002234205688869395946, 0.002642726781025562990, 0.003051247873181730033, 0.003459768965337897077, 0.003868290057494064120, 0.004685332241806398207 ),
 ( 0.000000000000000000, 1.000000000000000000 ),
 .UNSPECIFIED. ) 
 GEOMETRIC_REPRESENTATION_ITEM ( )  RATIONAL_B_SPLINE_SURFACE ( (
 ( 1.000000000000000000, 0.7071067811865475727, 1.000000000000000000),
 ( 1.000000000000000000, 0.7218508617830416974, 1.000000000000000000),
 ( 1.000000000000000000, 0.7387008909037698912, 1.000000000000000000),
 ( 1.000000000000000000, 0.7647615808955466887, 1.000000000000000000),
 ( 1.000000000000000000, 0.7734065576773528905, 1.000000000000000000),
 ( 1.000000000000000000, 0.7903558204260753284, 1.000000000000000000),
 ( 1.000000000000000000, 0.7987454157989255510, 1.000000000000000000),
 ( 1.000000000000000000, 0.8144265709895797123, 1.000000000000000000),
 ( 1.000000000000000000, 0.8216999247151044461, 1.000000000000000000),
 ( 1.000000000000000000, 0.8348485599609545282, 1.000000000000000000),
 ( 1.000000000000000000, 0.8407795038257930287, 1.000000000000000000),
 ( 1.000000000000000000, 0.8552130772089094890, 1.000000000000000000),
 ( 1.000000000000000000, 0.8606507091654866937, 1.000000000000000000),
 ( 1.000000000000000000, 0.8606282562001421610, 1.000000000000000000) ) ) 
 REPRESENTATION_ITEM ( '' )  SURFACE ( )  );
#2038=DIRECTION ( 'NONE',  ( -1.000000000000000000, 0.000000000000000000, 0.000000000000000000 ) ) ;
#2051=DIRECTION ( 'NONE',  ( -0.6727821148276317276, 0.7398406760702329610, 0.000000000000000000 ) ) ;
#2053=DIRECTION ( 'NONE',  ( -0.8746197071345569451, 0.4848096202550666312, 0.000000000000000000 ) ) ;
#2059=EDGE_LOOP ( 'NONE', ( #10542, #7788, #6445, #7214 ) ) ;
#2070=CARTESIAN_POINT ( 'NONE',  ( 56.56161818778031858, -7.613266777470379942, 48.51982618741349285 ) ) ;
#2075=ORIENTED_EDGE ( 'NONE', *, *, #8292, .T. ) ;
#2077=CARTESIAN_POINT ( 'NONE',  ( 69.45172263401887847, -2.801098317861658860, 76.51381904750685692 ) ) ;
#2081=CARTESIAN_POINT ( 'NONE',  ( 64.64681977576810823, -12.79380737173441140, 82.40005259842790508 ) ) ;
#2085=ORIENTED_EDGE ( 'NONE', *, *, #1603, .F. ) ;
#2088=DIRECTION ( 'NONE',  ( -0.8746197071345542806, 0.4848096202550715161, 0.000000000000000000 ) ) ;
#2089=CARTESIAN_POINT ( 'NONE',  ( 55.86211336638498182, 2.337731330496643167, 62.84860122826521689 ) ) ;
#2093=CARTESIAN_POINT ( 'NONE',  ( 71.64423341085262109, -14.38582895075278500, 71.19766410831374515 ) ) ;
#2103=ORIENTED_EDGE ( 'NONE', *, *, #14824, .T. ) ;
#2106=LINE ( 'NONE', #3423, #13928 ) ;
#2107=ADVANCED_FACE ( 'NONE', ( #12826 ), #8361, .T. ) ;
#2133=AXIS2_PLACEMENT_3D ( 'NONE', #10506, #11334, #6803 ) ;
#2140=TOROIDAL_SURFACE ( 'NONE', #3376, 2.000000000000000000, 1.000000000000000000 ) ;
#2143=ORIENTED_EDGE ( 'NONE', *, *, #11339, .F. ) ;
#2145=AXIS2_PLACEMENT_3D ( 'NONE', #5091, #2927, #9940 ) ;
#2155=CARTESIAN_POINT ( 'NONE',  ( 52.94134894379979528, -2.395505968190773327, 60.61639468829817190 ) ) ;
#2159=AXIS2_PLACEMENT_3D ( 'NONE', #5681, #12522, #8822 ) ;
#2176=DIRECTION ( 'NONE',  ( 0.1784957649143742442, 0.9839406800755992055, 8.214872995831076759E-16 ) ) ;
#2179=CARTESIAN_POINT ( 'NONE',  ( 70.26445833701072274, -4.474174595298148205, 76.19766410831374515 ) ) ;
#2180=VERTEX_POINT ( 'NONE', #2505 ) ;
#2182=VERTEX_POINT ( 'NONE', #14700 ) ;
#2188=ORIENTED_EDGE ( 'NONE', *, *, #8807, .F. ) ;
#2194=CIRCLE ( 'NONE', #14254, 7.924024642120691908 ) ;
#2195=DIRECTION ( 'NONE',  ( 0.000000000000000000, 0.000000000000000000, -1.000000000000000000 ) ) ;
#2199=EDGE_CURVE ( 'NONE', #612, #6287, #1439, .T. ) ;
#2200=DIRECTION ( 'NONE',  ( -0.000000000000000000, 0.000000000000000000, -1.000000000000000000 ) ) ;
#2205=DIRECTION ( 'NONE',  ( -0.09874083311360634663, -0.9951131834500188678, 0.000000000000000000 ) ) ;
#2209=DIRECTION ( 'NONE',  ( -0.8746197071345643836, 0.4848096202550529754, 0.000000000000000000 ) ) ;
#2212=ORIENTED_EDGE ( 'NONE', *, *, #6687, .F. ) ;
#2217=EDGE_CURVE ( 'NONE', #7606, #996, #6616, .T. ) ;
#2224=EDGE_LOOP ( 'NONE', ( #13942, #3623 ) ) ;
#2230=CARTESIAN_POINT ( 'NONE',  ( 58.44010239582257071, -7.290881550929530164, 48.51982618741349285 ) ) ;
#2235=FACE_OUTER_BOUND ( 'NONE', #6692, .T. ) ;
#2238=CARTESIAN_POINT ( 'NONE',  ( 69.40800899368780108, -3.479222266747031611, 72.26800456963103159 ) ) ;
#2242=DIRECTION ( 'NONE',  ( -0.6560590289829806299, 0.7547095802293147804, 0.000000000000000000 ) ) ;
#2243=AXIS2_PLACEMENT_3D ( 'NONE', #2970, #11412, #4108 ) ;
#2245=DIRECTION ( 'NONE',  ( -0.4643268659472232773, 0.8856639100469372305, 0.000000000000000000 ) ) ;
#2247=ORIENTED_EDGE ( 'NONE', *, *, #14497, .T. ) ;
#2256=EDGE_CURVE ( 'NONE', #117, #5924, #1680, .T. ) ;
#2263=EDGE_CURVE ( 'NONE', #3976, #1585, #10124, .T. ) ;
#2270=DIRECTION ( 'NONE',  ( 0.8746197071345569451, -0.4848096202550666312, 0.000000000000000000 ) ) ;
#2271=ADVANCED_FACE ( 'NONE', ( #14849 ), #5690, .F. ) ;
#2272=DIRECTION ( 'NONE',  ( -0.8208219420614786266, 0.4549890321264269955, 0.3453061251629919726 ) ) ;
#2282=AXIS2_PLACEMENT_3D ( 'NONE', #5396, #1078, #15167 ) ;
#2289=CARTESIAN_POINT ( 'NONE',  ( 65.43033136287209572, -11.84255085238262239, 75.82650736395967783 ) ) ;
#2295=CIRCLE ( 'NONE', #14099, 0.7892041907098263920 ) ;
#2300=ORIENTED_EDGE ( 'NONE', *, *, #13178, .F. ) ;
#2305=EDGE_LOOP ( 'NONE', ( #5018, #6461, #12046, #15107 ) ) ;
#2311=EDGE_CURVE ( 'NONE', #5234, #5320, #10285, .T. ) ;
#2313=CARTESIAN_POINT ( 'NONE',  ( 70.22960284859030367, -4.171102088227923943, 72.22139444149645726 ) ) ;
#2316=CARTESIAN_POINT ( 'NONE',  ( 65.33156958335074194, -11.86885053332497897, 72.68159868446096539 ) ) ;
#2317=DIRECTION ( 'NONE',  ( 0.8746197071345572782, -0.4848096202550659650, 0.000000000000000000 ) ) ;
#2320=CARTESIAN_POINT ( 'NONE',  ( 52.72354942432796321, 0.2729788054883388049, 60.61639468829817190 ) ) ;
#2321=EDGE_LOOP ( 'NONE', ( #4204, #5930, #4129, #14661 ) ) ;
#2324=EDGE_CURVE ( 'NONE', #1587, #2576, #14046, .T. ) ;
#2333=CARTESIAN_POINT ( 'NONE',  ( 71.78261302649870856, -15.60588809212342554, 75.19766410831374515 ) ) ;
#2338=DIRECTION ( 'NONE',  ( 0.3020115420618247892, -0.1674077314120183957, 0.9384901064608620613 ) ) ;
#2340=ORIENTED_EDGE ( 'NONE', *, *, #2851, .T. ) ;
#2343=ORIENTED_EDGE ( 'NONE', *, *, #12258, .T. ) ;
#2346=CARTESIAN_POINT ( 'NONE',  ( 55.86211336638498182, 2.337731330496643167, 60.61639468829817190 ) ) ;
#2349=LINE ( 'NONE', #11735, #9871 ) ;
#2361=VERTEX_POINT ( 'NONE', #14930 ) ;
#2362=CARTESIAN_POINT ( 'NONE',  ( 65.06009362424826747, -11.28293442697746940, 77.00361647515762797 ) ) ;
#2367=EDGE_CURVE ( 'NONE', #6435, #6563, #11574, .T. ) ;
#2370=DIRECTION ( 'NONE',  ( 0.3020115420618285085, -0.1674077314120178406, 0.9384901064608609511 ) ) ;
#2374=CIRCLE ( 'NONE', #8282, 0.7892041907098270581 ) ;
#2379=VERTEX_POINT ( 'NONE', #11851 ) ;
#2384=DIRECTION ( 'NONE',  ( 0.8746197071345569451, -0.4848096202550666312, 0.000000000000000000 ) ) ;
#2385=AXIS2_PLACEMENT_3D ( 'NONE', #14289, #10909, #11971 ) ;
#2386=LINE ( 'NONE', #2545, #9150 ) ;
#2394=CARTESIAN_POINT ( 'NONE',  ( 69.45589098779524306, -2.735193918331309870, 71.93997759770256550 ) ) ;
#2427=CARTESIAN_POINT ( 'NONE',  ( 69.40245686127688884, -3.447530338075270429, 77.00271947736730738 ) ) ;
#2429=DIRECTION ( 'NONE',  ( 0.000000000000000000, 0.000000000000000000, -1.000000000000000000 ) ) ;
#2435=ORIENTED_EDGE ( 'NONE', *, *, #6409, .F. ) ;
#2438=ORIENTED_EDGE ( 'NONE', *, *, #6065, .T. ) ;
#2439=CARTESIAN_POINT ( 'NONE',  ( 65.14189293393786784, -11.91678108959769489, 75.33440516864469316 ) ) ;
#2441=CARTESIAN_POINT ( 'NONE',  ( 61.18622467607353599, 2.299242679852278481, 54.56811043785582882 ) ) ;
#2453=EDGE_CURVE ( 'NONE', #1998, #13307, #7412, .T. ) ;
#2454=ORIENTED_EDGE ( 'NONE', *, *, #10449, .F. ) ;
#2455=ORIENTED_EDGE ( 'NONE', *, *, #8388, .T. ) ;
#2458=EDGE_CURVE ( 'NONE', #2379, #11350, #10854, .T. ) ;
#2459=EDGE_CURVE ( 'NONE', #10521, #13525, #1232, .T. ) ;
#2466=CARTESIAN_POINT ( 'NONE',  ( 69.98395955059181972, -3.185411745657274807, 73.04578369025026063 ) ) ;
#2467=ORIENTED_EDGE ( 'NONE', *, *, #10407, .F. ) ;
#2473=CARTESIAN_POINT ( 'NONE',  ( 65.92402464212069901, -2.249290599286308368, 47.51982618741348574 ) ) ;
#2477=ORIENTED_EDGE ( 'NONE', *, *, #5683, .T. ) ;
#2482=DIRECTION ( 'NONE',  ( 0.8746197071345572782, -0.4848096202550659650, 0.000000000000000000 ) ) ;
#2489=VECTOR ( 'NONE', #2506, 1000.000000000000000 ) ;
#2490=CARTESIAN_POINT ( 'NONE',  ( 118.5627027169299765, -35.81974489651393156, 54.40673322733725570 ) ) ;
#2493=DIRECTION ( 'NONE',  ( -0.000000000000000000, 0.000000000000000000, -1.000000000000000000 ) ) ;
#2495=DIRECTION ( 'NONE',  ( -0.000000000000000000, 0.000000000000000000, -1.000000000000000000 ) ) ;
#2502=AXIS2_PLACEMENT_3D ( 'NONE', #2, #13159, #13015 ) ;
#2504=AXIS2_PLACEMENT_3D ( 'NONE', #1500, #15143, #12999 ) ;
#2505=CARTESIAN_POINT ( 'NONE',  ( 69.46454297106444642, -2.294433322023680333, 73.19766410831374515 ) ) ;
#2506=DIRECTION ( 'NONE',  ( 0.8746197071345572782, -0.4848096202550659650, 0.000000000000000000 ) ) ;
#2512=CIRCLE ( 'NONE', #11105, 0.7892041907098270581 ) ;
#2515=CIRCLE ( 'NONE', #2994, 0.7892041907098261699 ) ;
#2518=CARTESIAN_POINT ( 'NONE',  ( 64.61411691698715742, -11.63232580666084104, 75.28919665560597707 ) ) ;
#2519=DIRECTION ( 'NONE',  ( 0.000000000000000000, 0.000000000000000000, -1.000000000000000000 ) ) ;
#2526=AXIS2_PLACEMENT_3D ( 'NONE', #13790, #3248, #13716 ) ;
#2527=DIRECTION ( 'NONE',  ( 0.8746197071345570562, -0.4848096202550665756, 0.000000000000000000 ) ) ;
#2531=ORIENTED_EDGE ( 'NONE', *, *, #242, .T. ) ;
#2532=CARTESIAN_POINT ( 'NONE',  ( 64.33396067855510125, -11.80593389191196962, 76.20215820740455115 ) ) ;
#2533=ORIENTED_EDGE ( 'NONE', *, *, #9628, .F. ) ;
#2545=CARTESIAN_POINT ( 'NONE',  ( 55.17185982823698964, 2.720345114498381012, 62.84860122826521689 ) ) ;
#2552=EDGE_LOOP ( 'NONE', ( #8864, #11402, #9965, #6153 ) ) ;
#2554=DIRECTION ( 'NONE',  ( 0.8746197071345569451, -0.4848096202550666312, 0.000000000000000000 ) ) ;
#2555=AXIS2_PLACEMENT_3D ( 'NONE', #2155, #11535, #5712 ) ;
#2557=DIRECTION ( 'NONE',  ( 0.3020115420618161295, -0.1674077314120152038, 0.9384901064608655030 ) ) ;
#2561=CYLINDRICAL_SURFACE ( 'NONE', #3136, 1.000000000000000888 ) ;
#2572=DIRECTION ( 'NONE',  ( 0.000000000000000000, 0.000000000000000000, -1.000000000000000000 ) ) ;
#2574=LINE ( 'NONE', #5257, #14780 ) ;
#2576=VERTEX_POINT ( 'NONE', #8612 ) ;
#2578=DIRECTION ( 'NONE',  ( -0.3020115420618249003, 0.1674077314120184790, -0.9384901064608621724 ) ) ;
#2579=CARTESIAN_POINT ( 'NONE',  ( 69.36597930231356202, -3.790285738762324108, 76.23203397659162306 ) ) ;
#2581=DIRECTION ( 'NONE',  ( -0.8208219420614786266, 0.4549890321264269399, 0.3453061251629920836 ) ) ;
#2591=DIRECTION ( 'NONE',  ( 0.000000000000000000, 0.000000000000000000, -1.000000000000000000 ) ) ;
#2599=ADVANCED_FACE ( 'NONE', ( #13526 ), #6308, .T. ) ;
#2606=AXIS2_PLACEMENT_3D ( 'NONE', #5493, #11472, #4400 ) ;
#2609=DIRECTION ( 'NONE',  ( -0.8746197071345569451, 0.4848096202550666312, 0.000000000000000000 ) ) ;
#2615=CARTESIAN_POINT ( 'NONE',  ( 52.50499674461036648, -3.053107681157296582, 60.61639468829817190 ) ) ;
#2621=EDGE_LOOP ( 'NONE', ( #4407, #5780, #6873, #3538 ) ) ;
#2623=CARTESIAN_POINT ( 'NONE',  ( 69.37830530362853665, -3.658688429576736123, 71.30420836299177267 ) ) ;
#2624=VECTOR ( 'NONE', #7150, 1000.000000000000000 ) ;
#2628=CYLINDRICAL_SURFACE ( 'NONE', #5345, 4.000000000000003553 ) ;
#2636=CIRCLE ( 'NONE', #6196, 1.000000000000000888 ) ;
#2640=CIRCLE ( 'NONE', #4847, 0.7892041907098276132 ) ;
#2641=DIRECTION ( 'NONE',  ( 0.8746197071345570562, -0.4848096202550662981, 0.000000000000000000 ) ) ;
#2643=CARTESIAN_POINT ( 'NONE',  ( 75.82472191495496361, -7.556279025088354473, 72.13615421477459222 ) ) ;
#2645=TOROIDAL_SURFACE ( 'NONE', #11231, 7.924024642120688355, 1.000000000000000000 ) ;
#2646=ORIENTED_EDGE ( 'NONE', *, *, #12807, .F. ) ;
#2650=ADVANCED_FACE ( 'NONE', ( #9782, #524 ), #14470, .F. ) ;
#2652=AXIS2_PLACEMENT_3D ( 'NONE', #11078, #607, #3927 ) ;
#2653=CARTESIAN_POINT ( 'NONE',  ( 69.46454297107186449, -2.294433320134092735, 75.47362438554114306 ) ) ;
#2655=CARTESIAN_POINT ( 'NONE',  ( 70.26445833701072274, -4.474174595298148205, 76.19766410831374515 ) ) ;
#2674=CARTESIAN_POINT ( 'NONE',  ( 71.64423341085262109, -14.38582895075279211, 71.19766410831374515 ) ) ;
#2697=CARTESIAN_POINT ( 'NONE',  ( 66.24916037665502699, -11.54047404292977319, 72.19766410831375936 ) ) ;
#2706=DIRECTION ( 'NONE',  ( -0.000000000000000000, 0.000000000000000000, -1.000000000000000000 ) ) ;
#2711=CARTESIAN_POINT ( 'NONE',  ( 58.00000000000000711, -2.249290599286309256, 87.40005259842790508 ) ) ;
#2713=CIRCLE ( 'NONE', #3446, 0.7892041907098303888 ) ;
#2718=CARTESIAN_POINT ( 'NONE',  ( 58.14816640453862107, 2.809303687574978614, 62.84860122826521689 ) ) ;
#2719=CARTESIAN_POINT ( 'NONE',  ( 70.02887381300654113, -3.323774946711823386, 75.65470943568233508 ) ) ;
#2723=CARTESIAN_POINT ( 'NONE',  ( 59.93923848102027563, 1.249188229251924742, 38.50000000000012790 ) ) ;
#2740=AXIS2_PLACEMENT_3D ( 'NONE', #2346, #12658, #2270 ) ;
#2743=FACE_OUTER_BOUND ( 'NONE', #156, .T. ) ;
#2755=DIRECTION ( 'NONE',  ( 0.000000000000000000, 0.000000000000000000, -1.000000000000000000 ) ) ;
#2759=ORIENTED_EDGE ( 'NONE', *, *, #14867, .T. ) ;
#2767=CIRCLE ( 'NONE', #11596, 10.46463184759104692 ) ;
#2770=VECTOR ( 'NONE', #12842, 999.9999999999998863 ) ;
#2774=EDGE_LOOP ( 'NONE', ( #11180, #3664, #14998, #5633 ) ) ;
#2777=ORIENTED_EDGE ( 'NONE', *, *, #2458, .F. ) ;
#2779=EDGE_CURVE ( 'NONE', #6596, #3976, #7893, .T. ) ;
#2783=FACE_OUTER_BOUND ( 'NONE', #2224, .T. ) ;
#2784=DIRECTION ( 'NONE',  ( -0.8746197071345569451, 0.4848096202550666312, 0.000000000000000000 ) ) ;
#2785=CARTESIAN_POINT ( 'NONE',  ( 68.02719294894561131, -7.807454411681058026, 77.19766410831374515 ) ) ;
#2802=VECTOR ( 'NONE', #9849, 1000.000000000000000 ) ;
#2810=ORIENTED_EDGE ( 'NONE', *, *, #6638, .T. ) ;
#2824=VERTEX_POINT ( 'NONE', #3348 ) ;
#2827=CYLINDRICAL_SURFACE ( 'NONE', #13768, 0.9999999999999957812 ) ;
#2828=ORIENTED_EDGE ( 'NONE', *, *, #10543, .F. ) ;
#2830=CARTESIAN_POINT ( 'NONE',  ( 52.42117158417902800, -3.175556148104785148, 60.61639468829817190 ) ) ;
#2832=ADVANCED_FACE ( 'NONE', ( #8048 ), #15128, .T. ) ;
#2836=FACE_OUTER_BOUND ( 'NONE', #9540, .T. ) ;
#2837=LINE ( 'NONE', #526, #13848 ) ;
#2842=ORIENTED_EDGE ( 'NONE', *, *, #7726, .T. ) ;
#2844=PLANE ( 'NONE',  #12726 ) ;
#2846=DIRECTION ( 'NONE',  ( -0.000000000000000000, 0.000000000000000000, -1.000000000000000000 ) ) ;
#2851=EDGE_CURVE ( 'NONE', #6117, #10912, #10666, .T. ) ;
#2854=AXIS2_PLACEMENT_3D ( 'NONE', #3382, #4535, #8079 ) ;
#2857=ORIENTED_EDGE ( 'NONE', *, *, #2851, .F. ) ;
#2860=DIRECTION ( 'NONE',  ( 0.000000000000000000, 0.000000000000000000, 1.000000000000000000 ) ) ;
#2865=CIRCLE ( 'NONE', #5089, 11.46463184759104870 ) ;
#2868=EDGE_CURVE ( 'NONE', #13763, #13591, #35, .T. ) ;
#2876=ORIENTED_EDGE ( 'NONE', *, *, #7691, .F. ) ;
#2878=DIRECTION ( 'NONE',  ( 0.8746197071345573892, -0.4848096202550657430, 0.000000000000000000 ) ) ;
#2884=CYLINDRICAL_SURFACE ( 'NONE', #6464, 1.000000000000000888 ) ;
#2886=EDGE_CURVE ( 'NONE', #8619, #3132, #2349, .T. ) ;
#2890=CIRCLE ( 'NONE', #11989, 0.9999999999999965583 ) ;
#2891=AXIS2_PLACEMENT_3D ( 'NONE', #5109, #14495, #8637 ) ;
#2893=CARTESIAN_POINT ( 'NONE',  ( 58.00000000000000711, -2.249290599286311032, -49.31370849898490150 ) ) ;
#2895=VERTEX_POINT ( 'NONE', #5904 ) ;
#2903=CARTESIAN_POINT ( 'NONE',  ( 69.43435019845104250, -3.089082358326208588, 71.61404092738268901 ) ) ;
#2908=ORIENTED_EDGE ( 'NONE', *, *, #15154, .F. ) ;
#2915=ADVANCED_FACE ( 'NONE', ( #4741 ), #12560, .F. ) ;
#2925=VERTEX_POINT ( 'NONE', #4660 ) ;
#2927=DIRECTION ( 'NONE',  ( -0.4848096202550659650, -0.8746197071345572782, -0.000000000000000000 ) ) ;
#2934=CARTESIAN_POINT ( 'NONE',  ( 64.71315123357256027, -11.54339494126895005, 71.67174403569786989 ) ) ;
#2943=DIRECTION ( 'NONE',  ( -0.8746197071345571672, 0.4848096202550659650, 0.000000000000000000 ) ) ;
#2945=( LENGTH_UNIT ( ) NAMED_UNIT ( * ) SI_UNIT ( .MILLI., .METRE. ) );
#2952=DIRECTION ( 'NONE',  ( 0.8208219420614786266, -0.4549890321264269955, -0.3453061251629919726 ) ) ;
#2953=AXIS2_PLACEMENT_3D ( 'NONE', #2490, #2338, #9346 ) ;
#2963=CIRCLE ( 'NONE', #4934, 0.9999999999999977796 ) ;
#2970=CARTESIAN_POINT ( 'NONE',  ( 61.57781019154727176, -5.828480965243416634, 62.84860122826521689 ) ) ;
#2974=DIRECTION ( 'NONE',  ( 1.000000000000000000, 0.000000000000000000, 0.000000000000000000 ) ) ;
#2977=AXIS2_PLACEMENT_3D ( 'NONE', #14523, #8672, #11055 ) ;
#2979=LINE ( 'NONE', #12367, #6410 ) ;
#2990=ORIENTED_EDGE ( 'NONE', *, *, #13123, .F. ) ;
#2994=AXIS2_PLACEMENT_3D ( 'NONE', #1991, #15008, #13699 ) ;
#3000=ORIENTED_EDGE ( 'NONE', *, *, #1099, .F. ) ;
#3004=VECTOR ( 'NONE', #2493, 1000.000000000000000 ) ;
#3005=DIRECTION ( 'NONE',  ( 0.000000000000000000, -0.000000000000000000, 1.000000000000000000 ) ) ;
#3006=AXIS2_PLACEMENT_3D ( 'NONE', #14105, #7100, #11786 ) ;
#3012=CARTESIAN_POINT ( 'NONE',  ( 64.97177248905298086, -11.36467339961058443, 72.35795077993141433 ) ) ;
#3021=AXIS2_PLACEMENT_3D ( 'NONE', #3933, #7180, #1404 ) ;
#3033=FACE_OUTER_BOUND ( 'NONE', #4631, .T. ) ;
#3036=VERTEX_POINT ( 'NONE', #5265 ) ;
#3044=CARTESIAN_POINT ( 'NONE',  ( 60.40269930420516431, 2.204737408716291647, 62.84860122826521689 ) ) ;
#3050=ADVANCED_FACE ( 'NONE', ( #1795 ), #6488, .T. ) ;
#3052=ORIENTED_EDGE ( 'NONE', *, *, #5683, .F. ) ;
#3055=ORIENTED_EDGE ( 'NONE', *, *, #9895, .T. ) ;
#3059=CARTESIAN_POINT ( 'NONE',  ( 52.35373241494735197, -0.8423457118892125894, 60.61639468829817190 ) ) ;
#3070=CARTESIAN_POINT ( 'NONE',  ( 58.80593636315131079, 3.245402227105440129, 48.51982618741349285 ) ) ;
#3071=EDGE_LOOP ( 'NONE', ( #13368, #4254, #3209, #14024, #371 ) ) ;
#3074=ORIENTED_EDGE ( 'NONE', *, *, #7357, .T. ) ;
#3076=CARTESIAN_POINT ( 'NONE',  ( 72.26742264675378635, -14.73126838498887281, 75.19766410831374515 ) ) ;
#3081=CARTESIAN_POINT ( 'NONE',  ( 48.84742675818896629, 2.824063592853377269, 61.61639468829817190 ) ) ;
#3082=CARTESIAN_POINT ( 'NONE',  ( 69.45530162631038706, -2.717604841179691366, 76.41417248176652777 ) ) ;
#3086=CARTESIAN_POINT ( 'NONE',  ( 69.98312355368540238, -3.182969857497201183, 73.06092304798380610 ) ) ;
#3096=CARTESIAN_POINT ( 'NONE',  ( 53.41380296247595538, -0.1096349785133995947, 48.51982618741349285 ) ) ;
#3099=VERTEX_POINT ( 'NONE', #13875 ) ;
#3105=EDGE_CURVE ( 'NONE', #1762, #3899, #5647, .T. ) ;
#3107=ORIENTED_EDGE ( 'NONE', *, *, #4323, .T. ) ;
#3118=VECTOR ( 'NONE', #7275, 1000.000000000000000 ) ;
#3122=CIRCLE ( 'NONE', #11731, 0.7892041907098253928 ) ;
#3127=DIRECTION ( 'NONE',  ( 0.000000000000000000, 0.000000000000000000, 1.000000000000000000 ) ) ;
#3128=CARTESIAN_POINT ( 'NONE',  ( 69.36208556723036622, -3.784586871655906570, 71.26433199163157894 ) ) ;
#3132=VERTEX_POINT ( 'NONE', #5412 ) ;
#3136=AXIS2_PLACEMENT_3D ( 'NONE', #1243, #8182, #22 ) ;
#3148=VECTOR ( 'NONE', #15223, 1000.000000000000000 ) ;
#3157=ORIENTED_EDGE ( 'NONE', *, *, #11189, .F. ) ;
#3159=DIRECTION ( 'NONE',  ( 0.4848096202550659650, 0.8746197071345572782, 0.000000000000000000 ) ) ;
#3165=VERTEX_POINT ( 'NONE', #1093 ) ;
#3168=ADVANCED_FACE ( 'NONE', ( #9338 ), #11642, .T. ) ;
#3169=ADVANCED_FACE ( 'NONE', ( #179 ), #4874, .T. ) ;
#3170=DIRECTION ( 'NONE',  ( -0.000000000000000000, -0.000000000000000000, 1.000000000000000000 ) ) ;
#3185=CYLINDRICAL_SURFACE ( 'NONE', #1786, 0.7892041907098262810 ) ;
#3190=CARTESIAN_POINT ( 'NONE',  ( 120.9867508182053086, -31.44664636084115017, 54.40673322733725570 ) ) ;
#3203=ORIENTED_EDGE ( 'NONE', *, *, #13971, .F. ) ;
#3209=ORIENTED_EDGE ( 'NONE', *, *, #6230, .T. ) ;
#3211=ADVANCED_FACE ( 'NONE', ( #9420 ), #14188, .T. ) ;
#3217=VERTEX_POINT ( 'NONE', #2333 ) ;
#3232=CARTESIAN_POINT ( 'NONE',  ( 64.11356537587559501, -11.94785244090458853, 73.19766410831374515 ) ) ;
#3241=AXIS2_PLACEMENT_3D ( 'NONE', #13853, #14636, #5624 ) ;
#3247=DIRECTION ( 'NONE',  ( 0.8746197071345571672, -0.4848096202550660205, 0.000000000000000000 ) ) ;
#3248=DIRECTION ( 'NONE',  ( 0.000000000000000000, 0.000000000000000000, 1.000000000000000000 ) ) ;
#3251=AXIS2_PLACEMENT_3D ( 'NONE', #3958, #4028, #11119 ) ;
#3256=AXIS2_PLACEMENT_3D ( 'NONE', #233, #13011, #11916 ) ;
#3257=LINE ( 'NONE', #1094, #238 ) ;
#3265=EDGE_LOOP ( 'NONE', ( #7746, #11331, #9067, #13249 ) ) ;
#3271=DIRECTION ( 'NONE',  ( -0.000000000000000000, 0.000000000000000000, -1.000000000000000000 ) ) ;
#3272=AXIS2_PLACEMENT_3D ( 'NONE', #614, #8852, #9874 ) ;
#3277=CARTESIAN_POINT ( 'NONE',  ( 59.12196317473677709, -7.688259372168277928, 48.51982618741349285 ) ) ;
#3279=CIRCLE ( 'NONE', #2555, 0.7892041907098262810 ) ;
#3295=DIRECTION ( 'NONE',  ( -0.8746197071345571672, 0.4848096202550660205, 0.000000000000000000 ) ) ;
#3299=ORIENTED_EDGE ( 'NONE', *, *, #1321, .T. ) ;
#3313=CARTESIAN_POINT ( 'NONE',  ( 69.28051765693513175, -4.295678830383772961, 77.19766410831374515 ) ) ;
#3315=CARTESIAN_POINT ( 'NONE',  ( 55.08546260466144417, 2.477934215446290445, 48.51982618741349285 ) ) ;
#3316=ORIENTED_EDGE ( 'NONE', *, *, #10774, .T. ) ;
#3317=CARTESIAN_POINT ( 'NONE',  ( 70.26445833701072274, -4.474174595298147317, 72.19766410831373094 ) ) ;
#3318=EDGE_CURVE ( 'NONE', #3816, #14247, #11781, .T. ) ;
#3320=DIRECTION ( 'NONE',  ( 0.000000000000000000, 0.000000000000000000, 1.000000000000000000 ) ) ;
#3324=VERTEX_POINT ( 'NONE', #13181 ) ;
#3332=DIRECTION ( 'NONE',  ( -0.000000000000000000, 0.000000000000000000, -1.000000000000000000 ) ) ;
#3336=EDGE_LOOP ( 'NONE', ( #15179, #2343, #12257, #11325 ) ) ;
#3342=CARTESIAN_POINT ( 'NONE',  ( 58.00000000000000711, -2.249290599286309256, 61.61639468829817190 ) ) ;
#3343=EDGE_CURVE ( 'NONE', #11072, #14286, #6612, .T. ) ;
#3345=AXIS2_PLACEMENT_3D ( 'NONE', #4197, #6441, #4125 ) ;
#3348=CARTESIAN_POINT ( 'NONE',  ( 69.28051765693513175, -4.295678830383772961, 77.19766410831374515 ) ) ;
#3351=ADVANCED_FACE ( 'NONE', ( #1774 ), #8495, .T. ) ;
#3352=VERTEX_POINT ( 'NONE', #3857 ) ;
#3361=DIRECTION ( 'NONE',  ( 0.000000000000000000, 0.000000000000000000, -1.000000000000000000 ) ) ;
#3362=ADVANCED_FACE ( 'NONE', ( #10877 ), #1483, .T. ) ;
#3367=EDGE_LOOP ( 'NONE', ( #1946, #1168, #13352, #2300 ) ) ;
#3368=CIRCLE ( 'NONE', #13941, 0.7892041907098262810 ) ;
#3371=DIRECTION ( 'NONE',  ( 0.000000000000000000, 0.000000000000000000, 1.000000000000000000 ) ) ;
#3376=AXIS2_PLACEMENT_3D ( 'NONE', #2674, #9379, #7368 ) ;
#3379=VERTEX_POINT ( 'NONE', #7483 ) ;
#3380=VERTEX_POINT ( 'NONE', #1701 ) ;
#3382=CARTESIAN_POINT ( 'NONE',  ( 48.84742675818896629, 2.824063592853376381, 81.40005259842790508 ) ) ;
#3391=CARTESIAN_POINT ( 'NONE',  ( 68.02719294894561131, -7.807454411681058026, 71.19766410831374515 ) ) ;
#3393=ORIENTED_EDGE ( 'NONE', *, *, #9079, .F. ) ;
#3394=ADVANCED_FACE ( 'NONE', ( #4070 ), #8586, .T. ) ;
#3395=DIRECTION ( 'NONE',  ( 0.000000000000000000, 0.000000000000000000, 1.000000000000000000 ) ) ;
#3397=CARTESIAN_POINT ( 'NONE',  ( 54.86190032082818391, 1.721056973166403603, 62.84860122826521689 ) ) ;
#3409=EDGE_CURVE ( 'NONE', #11544, #2824, #8451, .T. ) ;
#3420=CARTESIAN_POINT ( 'NONE',  ( 63.00747169918385993, -1.516790343742004055, 60.61639468829817190 ) ) ;
#3422=DIRECTION ( 'NONE',  ( -0.000000000000000000, -0.000000000000000000, 1.000000000000000000 ) ) ;
#3423=CARTESIAN_POINT ( 'NONE',  ( 63.36453054171181520, -0.8129776999179910701, 54.56811043785582882 ) ) ;
#3432=FACE_OUTER_BOUND ( 'NONE', #2305, .T. ) ;
#3433=EDGE_LOOP ( 'NONE', ( #11880, #2842, #1075, #5672 ) ) ;
#3436=EDGE_CURVE ( 'NONE', #2361, #4051, #9080, .T. ) ;
#3437=ORIENTED_EDGE ( 'NONE', *, *, #4601, .T. ) ;
#3439=AXIS2_PLACEMENT_3D ( 'NONE', #4970, #9680, #6416 ) ;
#3446=AXIS2_PLACEMENT_3D ( 'NONE', #10843, #4918, #1601 ) ;
#3455=B_SPLINE_CURVE_WITH_KNOTS ( 'NONE', 3,
 ( #1447, #5062, #144, #1217, #7373, #13074, #7220, #10610, #11832, #4990, #2532, #14152, #9767, #3901, #1526, #4833 ),
 .UNSPECIFIED., .F., .F.,
 ( 4, 2, 2, 2, 2, 2, 2, 4 ),
 ( 0.000000000000000000, 0.0003911934542035904491, 0.0007823869084071808982, 0.001173580362610771293, 0.001564773816814361796, 0.002347160725221542586, 0.002738354179425113791, 0.003129547633628685429 ),
 .UNSPECIFIED. ) ;
#3463=ORIENTED_EDGE ( 'NONE', *, *, #1321, .F. ) ;
#3469=CARTESIAN_POINT ( 'NONE',  ( 64.30331578579614416, -11.82577336004862545, 72.28357345370125131 ) ) ;
#3470=DIRECTION ( 'NONE',  ( 0.000000000000000000, 0.000000000000000000, 1.000000000000000000 ) ) ;
#3478=CIRCLE ( 'NONE', #2740, 0.7892041907098262810 ) ;
#3479=VECTOR ( 'NONE', #13091, 1000.000000000000000 ) ;
#3481=LINE ( 'NONE', #1088, #13098 ) ;
#3482=ORIENTED_EDGE ( 'NONE', *, *, #8846, .T. ) ;
#3487=CARTESIAN_POINT ( 'NONE',  ( 58.00000000000000711, -2.249290599286309256, 61.61639468829817190 ) ) ;
#3490=TOROIDAL_SURFACE ( 'NONE', #12090, 10.46463184759104870, 1.000000000000000000 ) ;
#3493=CARTESIAN_POINT ( 'NONE',  ( 52.94134894379979528, -2.395505968190773327, 62.84860122826521689 ) ) ;
#3495=VERTEX_POINT ( 'NONE', #11875 ) ;
#3500=ORIENTED_EDGE ( 'NONE', *, *, #4527, .T. ) ;
#3501=VECTOR ( 'NONE', #4551, 1000.000000000000000 ) ;
#3520=DIRECTION ( 'NONE',  ( 0.000000000000000000, 0.000000000000000000, 1.000000000000000000 ) ) ;
#3521=ORIENTED_EDGE ( 'NONE', *, *, #12529, .F. ) ;
#3522=VERTEX_POINT ( 'NONE', #7782 ) ;
#3531=DIRECTION ( 'NONE',  ( 0.8746197071345569451, -0.4848096202550666312, 0.000000000000000000 ) ) ;
#3538=ORIENTED_EDGE ( 'NONE', *, *, #5966, .F. ) ;
#3543=CARTESIAN_POINT ( 'NONE',  ( 70.25075679858845490, -4.321368936292105722, 72.19766410831378778 ) ) ;
#3547=CARTESIAN_POINT ( 'NONE',  ( 53.11142512232702018, -3.558169932106523881, 48.51982618741349285 ) ) ;
#3550=ORIENTED_EDGE ( 'NONE', *, *, #8348, .T. ) ;
#3551=CARTESIAN_POINT ( 'NONE',  ( 70.07302182237089028, -3.466915550704995574, 72.56882085266767035 ) ) ;
#3554=CYLINDRICAL_SURFACE ( 'NONE', #6306, 0.7892041907098262810 ) ;
#3567=CARTESIAN_POINT ( 'NONE',  ( 58.00000000000000711, -2.249290599286309256, 82.40005259842790508 ) ) ;
#3573=DIRECTION ( 'NONE',  ( -0.000000000000000000, -0.000000000000000000, -1.000000000000000000 ) ) ;
#3577=CARTESIAN_POINT ( 'NONE',  ( 38.50596956614688082, 13.12984319126714361, 91.03215601016300695 ) ) ;
#3585=LINE ( 'NONE', #14283, #3118 ) ;
#3588=ORIENTED_EDGE ( 'NONE', *, *, #5413, .F. ) ;
#3590=CARTESIAN_POINT ( 'NONE',  ( 65.33612023310359973, -11.06260784524912566, 77.14732870129599007 ) ) ;
#3593=AXIS2_PLACEMENT_3D ( 'NONE', #5262, #9959, #2952 ) ;
#3598=DIRECTION ( 'NONE',  ( -0.4848096202550659650, -0.8746197071345572782, 0.000000000000000000 ) ) ;
#3611=DIRECTION ( 'NONE',  ( -0.000000000000000000, 0.000000000000000000, -1.000000000000000000 ) ) ;
#3613=CIRCLE ( 'NONE', #12203, 0.7892041907098277242 ) ;
#3615=CIRCLE ( 'NONE', #2385, 8.924024642120691908 ) ;
#3616=CARTESIAN_POINT ( 'NONE',  ( 69.97972559857383601, -3.172990593254279457, 73.12044561456595204 ) ) ;
#3623=ORIENTED_EDGE ( 'NONE', *, *, #9810, .T. ) ;
#3627=CIRCLE ( 'NONE', #1657, 11.46463184759105047 ) ;
#3629=VERTEX_POINT ( 'NONE', #3315 ) ;
#3631=CYLINDRICAL_SURFACE ( 'NONE', #11840, 0.7892041907098262810 ) ;
#3634=ORIENTED_EDGE ( 'NONE', *, *, #4950, .F. ) ;
#3638=AXIS2_PLACEMENT_3D ( 'NONE', #3749, #13145, #294 ) ;
#3641=VECTOR ( 'NONE', #4032, 999.9999999999998863 ) ;
#3642=AXIS2_PLACEMENT_3D ( 'NONE', #9047, #13737, #8888 ) ;
#3643=DIRECTION ( 'NONE',  ( -0.000000000000000000, 0.000000000000000000, -1.000000000000000000 ) ) ;
#3645=CARTESIAN_POINT ( 'NONE',  ( 65.92402464212069901, -2.249290599286308368, 48.51982618741349285 ) ) ;
#3650=LINE ( 'NONE', #6116, #5161 ) ;
#3652=ORIENTED_EDGE ( 'NONE', *, *, #8882, .F. ) ;
#3655=DIRECTION ( 'NONE',  ( -0.000000000000000000, 0.000000000000000000, -1.000000000000000000 ) ) ;
#3660=CARTESIAN_POINT ( 'NONE',  ( 64.53644791741625397, -11.66848863668225711, 71.88150916912064758 ) ) ;
#3664=ORIENTED_EDGE ( 'NONE', *, *, #13178, .T. ) ;
#3669=CARTESIAN_POINT ( 'NONE',  ( 65.52872014148834978, -10.89904965666429071, 77.19766409816131159 ) ) ;
#3671=DIRECTION ( 'NONE',  ( 0.000000000000000000, 0.000000000000000000, 1.000000000000000000 ) ) ;
#3679=ORIENTED_EDGE ( 'NONE', *, *, #691, .F. ) ;
#3684=DIRECTION ( 'NONE',  ( 0.000000000000000000, 0.000000000000000000, -1.000000000000000000 ) ) ;
#3686=DIRECTION ( 'NONE',  ( 0.000000000000000000, 0.000000000000000000, 1.000000000000000000 ) ) ;
#3691=LINE ( 'NONE', #9555, #14057 ) ;
#3705=DIRECTION ( 'NONE',  ( -0.3020115420618322832, 0.1674077314120233917, -0.9384901064608587307 ) ) ;
#3714=AXIS2_PLACEMENT_3D ( 'NONE', #4192, #5522, #2205 ) ;
#3722=DIRECTION ( 'NONE',  ( -0.000000000000000000, 0.000000000000000000, -1.000000000000000000 ) ) ;
#3724=AXIS2_PLACEMENT_3D ( 'NONE', #4647, #1024, #12815 ) ;
#3729=CARTESIAN_POINT ( 'NONE',  ( 58.00000000000000711, -2.249290599286309256, 47.51982618741348574 ) ) ;
#3739=CARTESIAN_POINT ( 'NONE',  ( 64.17477533520170141, -11.90904020766107863, 75.73640774255487429 ) ) ;
#3740=ORIENTED_EDGE ( 'NONE', *, *, #4287, .F. ) ;
#3749=CARTESIAN_POINT ( 'NONE',  ( 56.97758043373130477, 2.707118148285912795, 62.84860122826521689 ) ) ;
#3755=CARTESIAN_POINT ( 'NONE',  ( 53.27389963060701916, 0.6670697996139958175, 60.61639468829817190 ) ) ;
#3760=AXIS2_PLACEMENT_3D ( 'NONE', #4600, #13992, #3295 ) ;
#3763=VERTEX_POINT ( 'NONE', #1900 ) ;
#3764=CIRCLE ( 'NONE', #1563, 1.000000000000007550 ) ;
#3765=EDGE_CURVE ( 'NONE', #8760, #6117, #14050, .T. ) ;
#3766=DIRECTION ( 'NONE',  ( 0.000000000000000000, 0.000000000000000000, 1.000000000000000000 ) ) ;
#3770=DIRECTION ( 'NONE',  ( 0.000000000000000000, 0.000000000000000000, 1.000000000000000000 ) ) ;
#3777=ADVANCED_FACE ( 'NONE', ( #6747 ), #9152, .T. ) ;
#3778=ORIENTED_EDGE ( 'NONE', *, *, #13971, .T. ) ;
#3780=CARTESIAN_POINT ( 'NONE',  ( 69.46411667222970721, -2.361176089487651897, 72.68029919668498451 ) ) ;
#3791=CARTESIAN_POINT ( 'NONE',  ( 58.00000000000000711, -2.249290599286309256, 47.51982618741348574 ) ) ;
#3795=ORIENTED_EDGE ( 'NONE', *, *, #1702, .F. ) ;
#3800=CARTESIAN_POINT ( 'NONE',  ( 69.32914122552278968, -4.026102965549716473, 76.25794738303314091 ) ) ;
#3802=CARTESIAN_POINT ( 'NONE',  ( 65.14877301755252859, -11.22304129159406116, 72.23267415556578896 ) ) ;
#3803=DIRECTION ( 'NONE',  ( -1.000000000000000000, 0.000000000000000000, 0.000000000000000000 ) ) ;
#3806=DIRECTION ( 'NONE',  ( -0.4848096202550659650, -0.8746197071345572782, 0.000000000000000000 ) ) ;
#3816=VERTEX_POINT ( 'NONE', #6346 ) ;
#3828=EDGE_CURVE ( 'NONE', #9158, #3629, #5198, .T. ) ;
#3829=VECTOR ( 'NONE', #2846, 1000.000000000000000 ) ;
#3847=AXIS2_PLACEMENT_3D ( 'NONE', #11592, #1052, #8226 ) ;
#3848=CARTESIAN_POINT ( 'NONE',  ( 53.54504563787001814, -4.650271872399136086, 60.61639468829817190 ) ) ;
#3855=ADVANCED_FACE ( 'NONE', ( #7349, #1577 ), #5042, .F. ) ;
#3857=CARTESIAN_POINT ( 'NONE',  ( 55.08546260466144417, 2.477934215446290445, 60.61639468829817190 ) ) ;
#3861=CIRCLE ( 'NONE', #10259, 10.46463184759104692 ) ;
#3863=ADVANCED_FACE ( 'NONE', ( #11322 ), #786, .T. ) ;
#3871=FACE_OUTER_BOUND ( 'NONE', #8927, .T. ) ;
#3875=CARTESIAN_POINT ( 'NONE',  ( 69.45987574584773938, -2.588318118538463608, 76.22979495466215383 ) ) ;
#3876=CARTESIAN_POINT ( 'NONE',  ( 64.29082196272626959, -11.83396660969246561, 72.31276519526322488 ) ) ;
#3878=ADVANCED_FACE ( 'NONE', ( #12569 ), #10109, .T. ) ;
#3883=ORIENTED_EDGE ( 'NONE', *, *, #2263, .T. ) ;
#3887=DIRECTION ( 'NONE',  ( 1.000000000000000000, 0.000000000000000000, 0.000000000000000000 ) ) ;
#3899=VERTEX_POINT ( 'NONE', #6413 ) ;
#3901=CARTESIAN_POINT ( 'NONE',  ( 64.12508379658279978, -11.94061857445316477, 75.45956441370945811 ) ) ;
#3902=ORIENTED_EDGE ( 'NONE', *, *, #12062, .F. ) ;
#3915=LINE ( 'NONE', #13309, #4596 ) ;
#3916=CARTESIAN_POINT ( 'NONE',  ( 63.55816381239476698, 7.777902349659290948, 82.40005259842790508 ) ) ;
#3927=DIRECTION ( 'NONE',  ( -0.9528381992908617759, -0.3034787735116703522, 0.000000000000000000 ) ) ;
#3929=B_SPLINE_CURVE_WITH_KNOTS ( 'NONE', 3,
 ( #6271, #1642, #9817, #14500, #5038, #3876, #9671, #14206, #3660, #8640, #13048, #10732, #7422, #8358, #3943, #7267, #195, #13341 ),
 .UNSPECIFIED., .F., .F.,
 ( 4, 2, 2, 2, 2, 2, 2, 2, 4 ),
 ( 0.000000000000000000, 0.0003958370570530560847, 0.0007916741141061121693, 0.001187511171159168254, 0.001583348228212224339, 0.001979185285265280640, 0.002375022342318336508, 0.002770859399371392376, 0.003166696456424448677 ),
 .UNSPECIFIED. ) ;
#3933=CARTESIAN_POINT ( 'NONE',  ( 64.64681977576810823, -12.79380737173441140, 73.19766410831374515 ) ) ;
#3936=ORIENTED_EDGE ( 'NONE', *, *, #14969, .F. ) ;
#3940=CARTESIAN_POINT ( 'NONE',  ( 60.40269930420516431, 2.204737408716291647, 48.51982618741349285 ) ) ;
#3941=ADVANCED_FACE ( 'NONE', ( #8029 ), #5705, .T. ) ;
#3942=CARTESIAN_POINT ( 'NONE',  ( 53.04398595309534414, -1.224959495890951100, 48.51982618741349285 ) ) ;
#3943=CARTESIAN_POINT ( 'NONE',  ( 65.32355913535712943, -11.07082656745060234, 71.26415692744444641 ) ) ;
#3944=EDGE_CURVE ( 'NONE', #9712, #2379, #9877, .T. ) ;
#3945=ADVANCED_FACE ( 'NONE', ( #12894 ), #12730, .T. ) ;
#3954=DIRECTION ( 'NONE',  ( -0.000000000000000000, -0.000000000000000000, -1.000000000000000000 ) ) ;
#3958=CARTESIAN_POINT ( 'NONE',  ( 57.26556849154462725, -7.256479411572841265, 60.61639468829817190 ) ) ;
#3963=DIRECTION ( 'NONE',  ( -0.8746197071345569451, 0.4848096202550666312, 0.000000000000000000 ) ) ;
#3975=CARTESIAN_POINT ( 'NONE',  ( 65.13162939602317181, -11.91918766459985157, 75.19766410831374515 ) ) ;
#3976=VERTEX_POINT ( 'NONE', #2179 ) ;
#3977=CIRCLE ( 'NONE', #7678, 5.496540510819677650 ) ;
#3979=CARTESIAN_POINT ( 'NONE',  ( 65.13162939602317181, -11.91918766459985157, 72.19766410831374515 ) ) ;
#3981=AXIS2_PLACEMENT_3D ( 'NONE', #12190, #3954, #3887 ) ;
#3983=CIRCLE ( 'NONE', #11610, 0.9999999999999951150 ) ;
#4001=DIRECTION ( 'NONE',  ( -0.8571673007072465600, -0.5150380749015093240, 0.000000000000000000 ) ) ;
#4004=CIRCLE ( 'NONE', #9679, 0.7892041907098262810 ) ;
#4013=DIRECTION ( 'NONE',  ( 0.8746197071345590546, -0.4848096202550628009, 0.000000000000000000 ) ) ;
#4015=CYLINDRICAL_SURFACE ( 'NONE', #6555, 0.7892041907098262810 ) ;
#4028=DIRECTION ( 'NONE',  ( 0.000000000000000000, 0.000000000000000000, 1.000000000000000000 ) ) ;
#4032=DIRECTION ( 'NONE',  ( 0.8208219420614786266, -0.4549890321264269955, -0.3453061251629919726 ) ) ;
#4035=EDGE_CURVE ( 'NONE', #14995, #3495, #8870, .T. ) ;
#4036=DIRECTION ( 'NONE',  ( 0.000000000000000000, 0.000000000000000000, -1.000000000000000000 ) ) ;
#4040=EDGE_LOOP ( 'NONE', ( #7922, #13761, #4377, #4768 ) ) ;
#4041=EDGE_CURVE ( 'NONE', #6176, #9708, #1990, .T. ) ;
#4043=VERTEX_POINT ( 'NONE', #15113 ) ;
#4045=CARTESIAN_POINT ( 'NONE',  ( 69.41635813202618976, -3.305880236131207184, 71.46816610982854456 ) ) ;
#4046=ORIENTED_EDGE ( 'NONE', *, *, #4183, .T. ) ;
#4048=CARTESIAN_POINT ( 'NONE',  ( 58.44010239582257071, -7.290881550929530164, 62.84860122826521689 ) ) ;
#4051=VERTEX_POINT ( 'NONE', #6571 ) ;
#4053=DIRECTION ( 'NONE',  ( -0.8746197071345569451, 0.4848096202550666312, 0.000000000000000000 ) ) ;
#4055=LINE ( 'NONE', #13452, #8558 ) ;
#4062=ORIENTED_EDGE ( 'NONE', *, *, #14035, .F. ) ;
#4065=CARTESIAN_POINT ( 'NONE',  ( 58.00000000000000711, -2.249290599286309256, 71.19766410831374515 ) ) ;
#4070=FACE_OUTER_BOUND ( 'NONE', #8352, .T. ) ;
#4075=ADVANCED_FACE ( 'NONE', ( #6648 ), #14654, .T. ) ;
#4082=CARTESIAN_POINT ( 'NONE',  ( 0.000000000000000000, 0.000000000000000000, 0.000000000000000000 ) ) ;
#4083=DIRECTION ( 'NONE',  ( -0.000000000000000000, -0.000000000000000000, 1.000000000000000000 ) ) ;
#4086=CIRCLE ( 'NONE', #14915, 3.999999999999996003 ) ;
#4092=EDGE_CURVE ( 'NONE', #2180, #2895, #7170, .T. ) ;
#4108=DIRECTION ( 'NONE',  ( -0.8746197071345569451, 0.4848096202550666312, 0.000000000000000000 ) ) ;
#4109=AXIS2_PLACEMENT_3D ( 'NONE', #724, #2200, #10131 ) ;
#4117=ORIENTED_EDGE ( 'NONE', *, *, #11909, .T. ) ;
#4120=EDGE_LOOP ( 'NONE', ( #11613, #3500, #4062, #1230 ) ) ;
#4124=DIRECTION ( 'NONE',  ( 0.8208219420614786266, -0.4549890321264268844, -0.3453061251629920281 ) ) ;
#4125=DIRECTION ( 'NONE',  ( 0.8746197071345569451, -0.4848096202550666312, 0.000000000000000000 ) ) ;
#4129=ORIENTED_EDGE ( 'NONE', *, *, #10653, .T. ) ;
#4132=EDGE_CURVE ( 'NONE', #8533, #3352, #3478, .T. ) ;
#4141=ORIENTED_EDGE ( 'NONE', *, *, #4763, .T. ) ;
#4144=ADVANCED_FACE ( 'NONE', ( #11572 ), #13072, .T. ) ;
#4150=EDGE_LOOP ( 'NONE', ( #5908, #10607, #13297, #279 ) ) ;
#4152=CARTESIAN_POINT ( 'NONE',  ( 64.96908986428803701, -11.35320032814772517, 71.45158253113490332 ) ) ;
#4156=VERTEX_POINT ( 'NONE', #43 ) ;
#4170=DIRECTION ( 'NONE',  ( 0.000000000000000000, 0.000000000000000000, 1.000000000000000000 ) ) ;
#4183=EDGE_CURVE ( 'NONE', #6287, #12282, #13553, .T. ) ;
#4192=CARTESIAN_POINT ( 'NONE',  ( 63.04142083571589694, -2.691337429055927988, 48.51982618741349285 ) ) ;
#4197=CARTESIAN_POINT ( 'NONE',  ( 55.86211336638498182, 2.337731330496643167, 60.61639468829817190 ) ) ;
#4199=CARTESIAN_POINT ( 'NONE',  ( 50.07597535787931520, -2.249290599286308368, 39.50000000000012790 ) ) ;
#4204=ORIENTED_EDGE ( 'NONE', *, *, #10943, .F. ) ;
#4216=ORIENTED_EDGE ( 'NONE', *, *, #9100, .T. ) ;
#4219=AXIS2_PLACEMENT_3D ( 'NONE', #6391, #14549, #6467 ) ;
#4224=ORIENTED_EDGE ( 'NONE', *, *, #8363, .T. ) ;
#4225=CARTESIAN_POINT ( 'NONE',  ( 58.00000000000000711, -2.249290599286309256, 48.51982618741349285 ) ) ;
#4234=CARTESIAN_POINT ( 'NONE',  ( 69.46221311397140141, -2.886128745360726278, 73.10613156102081689 ) ) ;
#4242=FACE_OUTER_BOUND ( 'NONE', #10497, .T. ) ;
#4254=ORIENTED_EDGE ( 'NONE', *, *, #12710, .F. ) ;
#4257=EDGE_LOOP ( 'NONE', ( #5302, #13233, #12869, #496, #1818 ) ) ;
#4287=EDGE_CURVE ( 'NONE', #8779, #1998, #3929, .T. ) ;
#4291=ORIENTED_EDGE ( 'NONE', *, *, #230, .F. ) ;
#4295=CARTESIAN_POINT ( 'NONE',  ( 68.90181265608016759, -8.292264031936127822, 72.19766410831374515 ) ) ;
#4298=ORIENTED_EDGE ( 'NONE', *, *, #5504, .T. ) ;
#4299=CARTESIAN_POINT ( 'NONE',  ( 65.05854647941774260, -11.28415211138448981, 71.39260873926113504 ) ) ;
#4301=LINE ( 'NONE', #13708, #6229 ) ;
#4303=ORIENTED_EDGE ( 'NONE', *, *, #3343, .F. ) ;
#4304=DIRECTION ( 'NONE',  ( 0.9816271834495682302, 0.1908089953667485572, 0.000000000000000000 ) ) ;
#4306=CARTESIAN_POINT ( 'NONE',  ( 63.43853564383336874, -3.373351419973840581, 48.51982618741349285 ) ) ;
#4308=ORIENTED_EDGE ( 'NONE', *, *, #1792, .F. ) ;
#4318=CARTESIAN_POINT ( 'NONE',  ( 71.64423341085262109, -14.38582895075279211, 72.19766410831374515 ) ) ;
#4323=EDGE_CURVE ( 'NONE', #14286, #1582, #10620, .T. ) ;
#4324=CIRCLE ( 'NONE', #9499, 3.999999999999994227 ) ;
#4340=CIRCLE ( 'NONE', #8301, 4.000000000000003553 ) ;
#4343=SPHERICAL_SURFACE ( 'NONE', #9694, 1.000000000000000000 ) ;
#4344=CIRCLE ( 'NONE', #421, 0.7892041907098322762 ) ;
#4347=CIRCLE ( 'NONE', #12975, 1.000000000000001998 ) ;
#4354=ORIENTED_EDGE ( 'NONE', *, *, #8670, .F. ) ;
#4362=AXIS2_PLACEMENT_3D ( 'NONE', #1695, #5021, #9725 ) ;
#4364=EDGE_CURVE ( 'NONE', #11220, #14748, #9887, .T. ) ;
#4365=CARTESIAN_POINT ( 'NONE',  ( 65.19224416878900286, -11.90459412701856756, 75.49439164730566176 ) ) ;
#4370=CIRCLE ( 'NONE', #12994, 0.7892041907098262810 ) ;
#4373=ORIENTED_EDGE ( 'NONE', *, *, #9488, .F. ) ;
#4374=CARTESIAN_POINT ( 'NONE',  ( 52.72873328492558187, -0.5014548242779810483, 48.51982618741349285 ) ) ;
#4377=ORIENTED_EDGE ( 'NONE', *, *, #3105, .F. ) ;
#4381=ORIENTED_EDGE ( 'NONE', *, *, #7447, .F. ) ;
#4382=EDGE_CURVE ( 'NONE', #13229, #7274, #2515, .T. ) ;
#4383=DIRECTION ( 'NONE',  ( -0.4848096202550659650, -0.8746197071345572782, 0.000000000000000000 ) ) ;
#4386=ORIENTED_EDGE ( 'NONE', *, *, #14867, .F. ) ;
#4388=CARTESIAN_POINT ( 'NONE',  ( 58.44010239582257071, -7.290881550929530164, 60.61639468829817190 ) ) ;
#4400=DIRECTION ( 'NONE',  ( 1.000000000000000000, 0.000000000000000000, 0.000000000000000000 ) ) ;
#4401=CARTESIAN_POINT ( 'NONE',  ( 54.03086304124234829, 0.8903401505190762233, 62.84860122826521689 ) ) ;
#4407=ORIENTED_EDGE ( 'NONE', *, *, #14824, .F. ) ;
#4416=CIRCLE ( 'NONE', #2953, 4.999999999999997335 ) ;
#4422=DIRECTION ( 'NONE',  ( 1.000000000000000000, 0.000000000000000000, 0.000000000000000000 ) ) ;
#4428=ORIENTED_EDGE ( 'NONE', *, *, #13345, .F. ) ;
#4430=ORIENTED_EDGE ( 'NONE', *, *, #691, .T. ) ;
#4434=CARTESIAN_POINT ( 'NONE',  ( 69.28051765693513175, -4.295678830383773850, 77.19766410831374515 ) ) ;
#4440=DIRECTION ( 'NONE',  ( 0.000000000000000000, 0.000000000000000000, 1.000000000000000000 ) ) ;
#4445=FACE_OUTER_BOUND ( 'NONE', #6405, .T. ) ;
#4448=ORIENTED_EDGE ( 'NONE', *, *, #11023, .F. ) ;
#4461=FACE_OUTER_BOUND ( 'NONE', #653, .T. ) ;
#4470=ORIENTED_EDGE ( 'NONE', *, *, #2256, .F. ) ;
#4472=FACE_OUTER_BOUND ( 'NONE', #9426, .T. ) ;
#4473=DIRECTION ( 'NONE',  ( 0.000000000000000000, 0.000000000000000000, 1.000000000000000000 ) ) ;
#4475=DIRECTION ( 'NONE',  ( 0.4848096202550659650, 0.8746197071345572782, 0.000000000000000000 ) ) ;
#4477=EDGE_LOOP ( 'NONE', ( #1338, #9932, #8605, #3652, #689 ) ) ;
#4488=ORIENTED_EDGE ( 'NONE', *, *, #9810, .F. ) ;
#4495=CIRCLE ( 'NONE', #3760, 10.46463184759104692 ) ;
#4497=CARTESIAN_POINT ( 'NONE',  ( 54.17164678268019173, 2.103670757168142114, 48.51982618741349285 ) ) ;
#4505=DIRECTION ( 'NONE',  ( 0.000000000000000000, 0.000000000000000000, 1.000000000000000000 ) ) ;
#4515=EDGE_CURVE ( 'NONE', #8533, #9158, #2386, .T. ) ;
#4523=CARTESIAN_POINT ( 'NONE',  ( 65.22735067928664421, -11.89594224596851468, 75.56344788988698724 ) ) ;
#4527=EDGE_CURVE ( 'NONE', #2895, #5118, #13468, .T. ) ;
#4532=DIRECTION ( 'NONE',  ( -0.8208219420614848438, 0.4549890321264155046, 0.3453061251629924167 ) ) ;
#4535=DIRECTION ( 'NONE',  ( -0.4848096202550659650, -0.8746197071345572782, -0.000000000000000000 ) ) ;
#4537=EDGE_CURVE ( 'NONE', #3899, #14177, #13016, .T. ) ;
#4544=ADVANCED_FACE ( 'NONE', ( #8245 ), #297, .T. ) ;
#4548=CARTESIAN_POINT ( 'NONE',  ( 69.40224406818397540, -3.449487665728846242, 71.39171174146984811 ) ) ;
#4549=CARTESIAN_POINT ( 'NONE',  ( 55.36337191871069763, -7.136966431295542534, 60.61639468829817190 ) ) ;
#4551=DIRECTION ( 'NONE',  ( -0.000000000000000000, 0.000000000000000000, -1.000000000000000000 ) ) ;
#4562=EDGE_CURVE ( 'NONE', #14878, #6522, #11336, .T. ) ;
#4569=EDGE_LOOP ( 'NONE', ( #8733, #7130, #2531, #9448 ) ) ;
#4572=ORIENTED_EDGE ( 'NONE', *, *, #9117, .T. ) ;
#4574=FACE_OUTER_BOUND ( 'NONE', #11764, .T. ) ;
#4578=LINE ( 'NONE', #13893, #13953 ) ;
#4580=DIRECTION ( 'NONE',  ( -0.4848096202550660205, -0.8746197071345573892, 0.000000000000000000 ) ) ;
#4586=CARTESIAN_POINT ( 'NONE',  ( 61.57781019154727176, -5.828480965243416634, 48.51982618741349285 ) ) ;
#4596=VECTOR ( 'NONE', #11001, 1000.000000000000000 ) ;
#4600=CARTESIAN_POINT ( 'NONE',  ( 58.00000000000000711, -2.249290599286309256, 82.40005259842790508 ) ) ;
#4601=EDGE_CURVE ( 'NONE', #3165, #8619, #8423, .T. ) ;
#4617=EDGE_CURVE ( 'NONE', #6145, #612, #2767, .T. ) ;
#4624=CARTESIAN_POINT ( 'NONE',  ( 72.24825649497627467, -14.72064441357683684, 73.07464432123546771 ) ) ;
#4626=AXIS2_PLACEMENT_3D ( 'NONE', #4401, #3643, #7104 ) ;
#4631=EDGE_LOOP ( 'NONE', ( #11438, #13264 ) ) ;
#4637=ORIENTED_EDGE ( 'NONE', *, *, #9454, .F. ) ;
#4645=DIRECTION ( 'NONE',  ( 0.8746197071345573892, -0.4848096202550657430, 0.000000000000000000 ) ) ;
#4647=CARTESIAN_POINT ( 'NONE',  ( 70.26445833701072274, -4.474174595298148205, 71.19766410831374515 ) ) ;
#4652=CYLINDRICAL_SURFACE ( 'NONE', #10749, 0.7892041907098262810 ) ;
#4654=DIRECTION ( 'NONE',  ( 0.000000000000000000, 0.000000000000000000, 1.000000000000000000 ) ) ;
#4660=CARTESIAN_POINT ( 'NONE',  ( 122.6668124272373745, -38.09469005714606737, 52.68020260152229639 ) ) ;
#4661=CARTESIAN_POINT ( 'NONE',  ( 63.36453054171181520, -0.8129776999179910701, 48.51982618741349285 ) ) ;
#4670=ORIENTED_EDGE ( 'NONE', *, *, #4562, .F. ) ;
#4671=CARTESIAN_POINT ( 'NONE',  ( 64.62474033849325394, -11.62473885758638303, 75.37908211999966568 ) ) ;
#4672=FACE_OUTER_BOUND ( 'NONE', #8334, .T. ) ;
#4679=LINE ( 'NONE', #9376, #3148 ) ;
#4684=DIRECTION ( 'NONE',  ( 0.8208219420614786266, -0.4549890321264268289, -0.3453061251629919726 ) ) ;
#4694=DIRECTION ( 'NONE',  ( 0.8746197071345571672, -0.4848096202550662981, 0.000000000000000000 ) ) ;
#4695=EDGE_LOOP ( 'NONE', ( #12254, #10078, #7711, #7351 ) ) ;
#4715=DIRECTION ( 'NONE',  ( 0.000000000000000000, 0.000000000000000000, -1.000000000000000000 ) ) ;
#4723=DIRECTION ( 'NONE',  ( -0.8208219420614786266, 0.4549890321264268289, 0.3453061251629919726 ) ) ;
#4724=AXIS2_PLACEMENT_3D ( 'NONE', #1380, #6086, #5936 ) ;
#4731=CYLINDRICAL_SURFACE ( 'NONE', #12336, 8.924024642120684803 ) ;
#4732=VECTOR ( 'NONE', #8093, 1000.000000000000000 ) ;
#4734=DIRECTION ( 'NONE',  ( 0.8746197071345569451, -0.4848096202550666312, 0.000000000000000000 ) ) ;
#4741=FACE_OUTER_BOUND ( 'NONE', #4477, .T. ) ;
#4754=CARTESIAN_POINT ( 'NONE',  ( 64.97069784687126059, -11.35197416150241523, 76.94490957099723971 ) ) ;
#4755=CARTESIAN_POINT ( 'NONE',  ( 58.00000000000000711, -2.249290599286309256, 81.40005259842790508 ) ) ;
#4758=ORIENTED_EDGE ( 'NONE', *, *, #667, .T. ) ;
#4762=ADVANCED_FACE ( 'NONE', ( #4242 ), #1933, .T. ) ;
#4763=EDGE_CURVE ( 'NONE', #3352, #11220, #14328, .T. ) ;
#4768=ORIENTED_EDGE ( 'NONE', *, *, #7999, .F. ) ;
#4774=FACE_OUTER_BOUND ( 'NONE', #6720, .T. ) ;
#4775=ORIENTED_EDGE ( 'NONE', *, *, #2324, .F. ) ;
#4785=CARTESIAN_POINT ( 'NONE',  ( 69.32502553878046569, -4.050333426515871693, 71.19766411846617871 ) ) ;
#4792=EDGE_LOOP ( 'NONE', ( #4935, #12146, #8015, #14909 ) ) ;
#4800=ORIENTED_EDGE ( 'NONE', *, *, #10449, .T. ) ;
#4804=CARTESIAN_POINT ( 'NONE',  ( 58.00000000000000711, -2.249290599286309256, 82.40005259842790508 ) ) ;
#4806=CARTESIAN_POINT ( 'NONE',  ( 62.88869237673507229, 0.3854521819929429549, 54.56811043785582882 ) ) ;
#4807=DIRECTION ( 'NONE',  ( -0.000000000000000000, 0.000000000000000000, -1.000000000000000000 ) ) ;
#4808=CARTESIAN_POINT ( 'NONE',  ( 70.17072936512437309, -3.859920535181831980, 76.07070489651268019 ) ) ;
#4813=CARTESIAN_POINT ( 'NONE',  ( 62.32645299789339788, 5.555837219666858395, 48.51982618741349285 ) ) ;
#4822=ORIENTED_EDGE ( 'NONE', *, *, #4041, .F. ) ;
#4823=CARTESIAN_POINT ( 'NONE',  ( 65.68066376434035192, -11.76402373953423819, 76.00162494909807265 ) ) ;
#4833=CARTESIAN_POINT ( 'NONE',  ( 64.11356537587559501, -11.94785244090458498, 75.19766410831374515 ) ) ;
#4835=DIRECTION ( 'NONE',  ( 0.8746197071345571672, -0.4848096202550662981, 0.000000000000000000 ) ) ;
#4840=( GEOMETRIC_REPRESENTATION_CONTEXT ( 3 ) GLOBAL_UNCERTAINTY_ASSIGNED_CONTEXT ( ( #8579 ) ) GLOBAL_UNIT_ASSIGNED_CONTEXT ( ( #854, #9101, #11632 ) ) REPRESENTATION_CONTEXT ( 'NONE', 'WORKASPACE' ) );
#4847=AXIS2_PLACEMENT_3D ( 'NONE', #7265, #1192, #10583 ) ;
#4848=CARTESIAN_POINT ( 'NONE',  ( 70.04947142428893869, -3.389475778999904598, 72.64451403610593161 ) ) ;
#4862=EDGE_CURVE ( 'NONE', #4043, #10980, #3983, .T. ) ;
#4867=AXIS2_PLACEMENT_3D ( 'NONE', #142, #3598, #10759 ) ;
#4868=DIRECTION ( 'NONE',  ( 0.000000000000000000, 0.000000000000000000, 1.000000000000000000 ) ) ;
#4870=CIRCLE ( 'NONE', #1423, 1.000000000000000888 ) ;
#4872=CIRCLE ( 'NONE', #5111, 0.9999999999999978906 ) ;
#4874=CYLINDRICAL_SURFACE ( 'NONE', #1213, 5.000000000000000000 ) ;
#4879=DIRECTION ( 'NONE',  ( -0.000000000000000000, -0.000000000000000000, 1.000000000000000000 ) ) ;
#4880=ORIENTED_EDGE ( 'NONE', *, *, #1759, .T. ) ;
#4881=CARTESIAN_POINT ( 'NONE',  ( 62.00000000000001421, -2.249290599286311032, 38.50000000000012790 ) ) ;
#4884=ORIENTED_EDGE ( 'NONE', *, *, #2453, .F. ) ;
#4886=DIRECTION ( 'NONE',  ( -0.4848096202550659650, -0.8746197071345572782, -0.000000000000000000 ) ) ;
#4888=CARTESIAN_POINT ( 'NONE',  ( 69.40811084813233833, -3.478390292315104659, 76.12692897370897072 ) ) ;
#4897=EDGE_CURVE ( 'NONE', #3324, #11072, #3481, .T. ) ;
#4901=CARTESIAN_POINT ( 'NONE',  ( 58.00000000000000711, -2.249290599286309256, 82.40005259842790508 ) ) ;
#4907=ADVANCED_FACE ( 'NONE', ( #23 ), #9412, .T. ) ;
#4909=DIRECTION ( 'NONE',  ( -0.000000000000000000, 0.000000000000000000, -1.000000000000000000 ) ) ;
#4918=DIRECTION ( 'NONE',  ( 0.000000000000000000, 0.000000000000000000, 1.000000000000000000 ) ) ;
#4926=DIRECTION ( 'NONE',  ( 0.000000000000000000, 0.000000000000000000, 1.000000000000000000 ) ) ;
#4930=DIRECTION ( 'NONE',  ( 0.6293203910575899673, 0.7771459614506929237, 0.000000000000000000 ) ) ;
#4932=CARTESIAN_POINT ( 'NONE',  ( 65.46435777888771668, -11.83269322980322968, 72.53932447423565577 ) ) ;
#4934=AXIS2_PLACEMENT_3D ( 'NONE', #12600, #7982, #2051 ) ;
#4935=ORIENTED_EDGE ( 'NONE', *, *, #9516, .F. ) ;
#4946=DIRECTION ( 'NONE',  ( -0.8208219420614781825, 0.4549890321264266069, 0.3453061251629932493 ) ) ;
#4950=EDGE_CURVE ( 'NONE', #5064, #5118, #1778, .T. ) ;
#4952=AXIS2_PLACEMENT_3D ( 'NONE', #12648, #6955, #5806 ) ;
#4953=AXIS2_PLACEMENT_3D ( 'NONE', #6169, #9714, #11922 ) ;
#4957=DIRECTION ( 'NONE',  ( 0.8746197071345571672, -0.4848096202550661871, 0.000000000000000000 ) ) ;
#4963=AXIS2_PLACEMENT_3D ( 'NONE', #10144, #14988, #13674 ) ;
#4965=CARTESIAN_POINT ( 'NONE',  ( 66.10060683232276801, -11.60666214070378111, 72.22272846899819854 ) ) ;
#4966=DIRECTION ( 'NONE',  ( -0.8746197071345573892, 0.4848096202550659650, 0.000000000000000000 ) ) ;
#4970=CARTESIAN_POINT ( 'NONE',  ( 61.36510378087922390, 1.530577915148011225, 60.61639468829817190 ) ) ;
#4978=CARTESIAN_POINT ( 'NONE',  ( 64.79775953413574996, -11.48183855866792058, 76.80558578852820517 ) ) ;
#4987=CIRCLE ( 'NONE', #3021, 0.9999999999999954481 ) ;
#4988=ORIENTED_EDGE ( 'NONE', *, *, #9193, .T. ) ;
#4990=CARTESIAN_POINT ( 'NONE',  ( 64.46078417747735045, -11.72191032465318195, 76.42234406089987431 ) ) ;
#4991=EDGE_CURVE ( 'NONE', #3132, #11072, #12848, .T. ) ;
#4999=AXIS2_PLACEMENT_3D ( 'NONE', #8231, #3371, #3531 ) ;
#5006=ORIENTED_EDGE ( 'NONE', *, *, #9720, .F. ) ;
#5009=DIRECTION ( 'NONE',  ( -0.2475627213817241101, 0.9688718692283695422, 0.000000000000000000 ) ) ;
#5017=DIRECTION ( 'NONE',  ( -0.000000000000000000, -0.000000000000000000, -1.000000000000000000 ) ) ;
#5018=ORIENTED_EDGE ( 'NONE', *, *, #1123, .F. ) ;
#5019=ADVANCED_FACE ( 'NONE', ( #7323 ), #12313, .T. ) ;
#5021=DIRECTION ( 'NONE',  ( 0.8208219420614786266, -0.4549890321264269399, -0.3453061251629919171 ) ) ;
#5025=EDGE_CURVE ( 'NONE', #2895, #1585, #7480, .T. ) ;
#5032=VERTEX_POINT ( 'NONE', #1478 ) ;
#5037=CARTESIAN_POINT ( 'NONE',  ( 69.97972559771834256, -3.172990592780090324, 75.33564424702136364 ) ) ;
#5038=CARTESIAN_POINT ( 'NONE',  ( 64.20414115715628611, -11.89030131877283480, 72.55252335815228548 ) ) ;
#5042=PLANE ( 'NONE',  #7411 ) ;
#5049=ORIENTED_EDGE ( 'NONE', *, *, #5859, .T. ) ;
#5052=FACE_OUTER_BOUND ( 'NONE', #713, .T. ) ;
#5056=PRODUCT_DEFINITION ( 'UNKNOWN', '', #5854, #9363 ) ;
#5062=CARTESIAN_POINT ( 'NONE',  ( 65.61547001893620745, -10.82016271803256657, 77.19766410831377357 ) ) ;
#5063=VERTEX_POINT ( 'NONE', #11227 ) ;
#5064=VERTEX_POINT ( 'NONE', #4295 ) ;
#5072=ORIENTED_EDGE ( 'NONE', *, *, #11516, .F. ) ;
#5083=ORIENTED_EDGE ( 'NONE', *, *, #4041, .T. ) ;
#5085=ORIENTED_EDGE ( 'NONE', *, *, #7153, .F. ) ;
#5089=AXIS2_PLACEMENT_3D ( 'NONE', #5915, #2591, #12050 ) ;
#5091=CARTESIAN_POINT ( 'NONE',  ( 76.14589960879430919, -7.734310727912411920, 75.19766410831374515 ) ) ;
#5103=AXIS2_PLACEMENT_3D ( 'NONE', #121, #4807, #268 ) ;
#5109=CARTESIAN_POINT ( 'NONE',  ( 9.211295467215947497, 29.36814620404575038, 73.19766410831374515 ) ) ;
#5110=CIRCLE ( 'NONE', #7078, 4.000000000000003553 ) ;
#5111=AXIS2_PLACEMENT_3D ( 'NONE', #8943, #3170, #2088 ) ;
#5118=VERTEX_POINT ( 'NONE', #5468 ) ;
#5131=DIRECTION ( 'NONE',  ( -0.8746197071345572782, 0.4848096202550659650, -0.000000000000000000 ) ) ;
#5137=ORIENTED_EDGE ( 'NONE', *, *, #12365, .T. ) ;
#5142=CYLINDRICAL_SURFACE ( 'NONE', #9764, 1.000000000000007550 ) ;
#5143=DIRECTION ( 'NONE',  ( 0.000000000000000000, 0.000000000000000000, 1.000000000000000000 ) ) ;
#5147=AXIS2_PLACEMENT_3D ( 'NONE', #11177, #861, #11553 ) ;
#5161=VECTOR ( 'NONE', #9662, 1000.000000000000000 ) ;
#5174=DIRECTION ( 'NONE',  ( -0.3020115420618247892, 0.1674077314120183957, -0.9384901064608620613 ) ) ;
#5175=CARTESIAN_POINT ( 'NONE',  ( 58.00000000000000711, -2.249290599286309256, 82.40005259842790508 ) ) ;
#5178=EDGE_CURVE ( 'NONE', #9615, #153, #7229, .T. ) ;
#5179=DIRECTION ( 'NONE',  ( 0.2135987722749887463, 0.9769214730379394140, 0.000000000000000000 ) ) ;
#5180=EDGE_CURVE ( 'NONE', #3352, #3629, #11689, .T. ) ;
#5185=ADVANCED_FACE ( 'NONE', ( #1301 ), #7001, .T. ) ;
#5190=EDGE_LOOP ( 'NONE', ( #5273, #9054, #5684, #8894, #13312, #12148 ) ) ;
#5197=ORIENTED_EDGE ( 'NONE', *, *, #4132, .T. ) ;
#5198=CIRCLE ( 'NONE', #2504, 0.7892041907098253928 ) ;
#5204=VECTOR ( 'NONE', #15089, 1000.000000000000000 ) ;
#5216=VECTOR ( 'NONE', #5835, 999.9999999999998863 ) ;
#5217=CARTESIAN_POINT ( 'NONE',  ( 65.13162939602317181, -11.91918766459985157, 73.19766410831374515 ) ) ;
#5220=AXIS2_PLACEMENT_3D ( 'NONE', #8074, #4532, #9307 ) ;
#5227=CYLINDRICAL_SURFACE ( 'NONE', #8540, 0.7892041907098262810 ) ;
#5228=DIRECTION ( 'NONE',  ( 0.000000000000000000, 0.000000000000000000, -1.000000000000000000 ) ) ;
#5230=EDGE_LOOP ( 'NONE', ( #7380, #7053, #5072, #5849 ) ) ;
#5234=VERTEX_POINT ( 'NONE', #11842 ) ;
#5241=EDGE_CURVE ( 'NONE', #2361, #2895, #15157, .T. ) ;
#5243=ADVANCED_FACE ( 'NONE', ( #12863 ), #6014, .F. ) ;
#5247=DIRECTION ( 'NONE',  ( -0.000000000000000000, 0.000000000000000000, -1.000000000000000000 ) ) ;
#5253=CARTESIAN_POINT ( 'NONE',  ( 69.46221311437309964, -2.886128739015261679, 73.19766410831374515 ) ) ;
#5257=CARTESIAN_POINT ( 'NONE',  ( 52.83848824477699679, -4.298675648159541396, 54.56811043785582882 ) ) ;
#5261=ORIENTED_EDGE ( 'NONE', *, *, #13873, .T. ) ;
#5262=CARTESIAN_POINT ( 'NONE',  ( 124.7888489864508728, -33.55418379006125917, 51.74171249506144932 ) ) ;
#5263=ORIENTED_EDGE ( 'NONE', *, *, #2779, .F. ) ;
#5265=CARTESIAN_POINT ( 'NONE',  ( 53.45023817967523172, -5.433760736713491468, 60.61639468829817190 ) ) ;
#5266=DIRECTION ( 'NONE',  ( 0.8746197071345569451, -0.4848096202550666312, 0.000000000000000000 ) ) ;
#5273=ORIENTED_EDGE ( 'NONE', *, *, #9971, .T. ) ;
#5282=DIRECTION ( 'NONE',  ( -0.000000000000000000, -0.000000000000000000, 1.000000000000000000 ) ) ;
#5283=EDGE_CURVE ( 'NONE', #12099, #11185, #11769, .T. ) ;
#5285=ADVANCED_FACE ( 'NONE', ( #4774 ), #13374, .T. ) ;
#5288=EDGE_LOOP ( 'NONE', ( #940, #8878, #1056, #1336 ) ) ;
#5297=ORIENTED_EDGE ( 'NONE', *, *, #1759, .F. ) ;
#5302=ORIENTED_EDGE ( 'NONE', *, *, #10466, .F. ) ;
#5307=EDGE_LOOP ( 'NONE', ( #15136, #9084, #13494, #12709 ) ) ;
#5316=CARTESIAN_POINT ( 'NONE',  ( 65.61367503392970946, -11.78584904878405304, 72.43470407172173964 ) ) ;
#5317=DIRECTION ( 'NONE',  ( 0.000000000000000000, 0.000000000000000000, -1.000000000000000000 ) ) ;
#5320=VERTEX_POINT ( 'NONE', #8744 ) ;
#5324=AXIS2_PLACEMENT_3D ( 'NONE', #6141, #2519, #10752 ) ;
#5325=DIRECTION ( 'NONE',  ( -0.000000000000000000, -0.000000000000000000, 1.000000000000000000 ) ) ;
#5327=VERTEX_POINT ( 'NONE', #2830 ) ;
#5328=EDGE_CURVE ( 'NONE', #14748, #8583, #9935, .T. ) ;
#5344=DIRECTION ( 'NONE',  ( -0.8746197071345569451, 0.4848096202550666312, 0.000000000000000000 ) ) ;
#5345=AXIS2_PLACEMENT_3D ( 'NONE', #9331, #15177, #393 ) ;
#5363=AXIS2_PLACEMENT_3D ( 'NONE', #7692, #7537, #11071 ) ;
#5370=EDGE_LOOP ( 'NONE', ( #13066, #10462, #7377, #1882, #15009, #2810, #7162 ) ) ;
#5371=EDGE_CURVE ( 'NONE', #9847, #13591, #11140, .T. ) ;
#5387=DIRECTION ( 'NONE',  ( 0.000000000000000000, 0.000000000000000000, -1.000000000000000000 ) ) ;
#5394=DIRECTION ( 'NONE',  ( -0.8746197071345576113, 0.4848096202550652434, 0.000000000000000000 ) ) ;
#5396=CARTESIAN_POINT ( 'NONE',  ( 118.5627027169299765, -35.81974489651393156, 54.40673322733726280 ) ) ;
#5399=LINE ( 'NONE', #9091, #11750 ) ;
#5401=CIRCLE ( 'NONE', #1950, 5.496540510819668768 ) ;
#5409=DIRECTION ( 'NONE',  ( 0.000000000000000000, 0.000000000000000000, 1.000000000000000000 ) ) ;
#5412=CARTESIAN_POINT ( 'NONE',  ( 55.36337191871069763, -7.136966431295542534, 48.51982618741349285 ) ) ;
#5413=EDGE_CURVE ( 'NONE', #8760, #11327, #453, .T. ) ;
#5436=AXIS2_PLACEMENT_3D ( 'NONE', #1219, #14081, #1293 ) ;
#5440=DIRECTION ( 'NONE',  ( -0.000000000000000000, 0.000000000000000000, -1.000000000000000000 ) ) ;
#5444=LINE ( 'NONE', #8904, #7290 ) ;
#5452=CARTESIAN_POINT ( 'NONE',  ( 65.35217890228821602, -11.86361580896913459, 75.75081418052154447 ) ) ;
#5456=CARTESIAN_POINT ( 'NONE',  ( 57.83740799265796539, -7.800393779465814248, 60.61639468829817190 ) ) ;
#5468=CARTESIAN_POINT ( 'NONE',  ( 70.26445833701072274, -4.474174595298148205, 72.19766410831374515 ) ) ;
#5475=CARTESIAN_POINT ( 'NONE',  ( 69.97972559857380759, -3.172990593254279457, 75.35198908857846334 ) ) ;
#5483=CIRCLE ( 'NONE', #3272, 0.7892041907098245046 ) ;
#5490=DIRECTION ( 'NONE',  ( -0.000000000000000000, 0.000000000000000000, -1.000000000000000000 ) ) ;
#5492=ORIENTED_EDGE ( 'NONE', *, *, #5180, .T. ) ;
#5493=CARTESIAN_POINT ( 'NONE',  ( -16.99999999999998579, -2.249290599286303927, -38.00000000000012079 ) ) ;
#5495=CIRCLE ( 'NONE', #7697, 4.000000000000003553 ) ;
#5498=CARTESIAN_POINT ( 'NONE',  ( 76.12673345701679750, -7.723686756500376838, 73.07464432123545350 ) ) ;
#5503=VERTEX_POINT ( 'NONE', #8823 ) ;
#5504=EDGE_CURVE ( 'NONE', #11327, #13149, #6514, .T. ) ;
#5505=DIRECTION ( 'NONE',  ( -0.8124228799517130284, 0.5830686615922384686, 0.000000000000000000 ) ) ;
#5508=VECTOR ( 'NONE', #13922, 1000.000000000000000 ) ;
#5514=DIRECTION ( 'NONE',  ( 0.000000000000000000, 0.000000000000000000, 1.000000000000000000 ) ) ;
#5517=FACE_OUTER_BOUND ( 'NONE', #6355, .T. ) ;
#5522=DIRECTION ( 'NONE',  ( 0.000000000000000000, 0.000000000000000000, 1.000000000000000000 ) ) ;
#5527=CARTESIAN_POINT ( 'NONE',  ( 69.46454297106444642, -2.294433322023680333, 73.19766410831374515 ) ) ;
#5535=DIRECTION ( 'NONE',  ( -0.000000000000000000, 0.000000000000000000, 1.000000000000000000 ) ) ;
#5536=ORIENTED_EDGE ( 'NONE', *, *, #4183, .F. ) ;
#5553=CARTESIAN_POINT ( 'NONE',  ( 69.44459735978651338, -3.127033676967585052, 72.52731926747081559 ) ) ;
#5558=ORIENTED_EDGE ( 'NONE', *, *, #12088, .F. ) ;
#5565=DIRECTION ( 'NONE',  ( 0.8746197071345573892, -0.4848096202550657430, 0.000000000000000000 ) ) ;
#5571=ORIENTED_EDGE ( 'NONE', *, *, #14502, .F. ) ;
#5572=ORIENTED_EDGE ( 'NONE', *, *, #1010, .T. ) ;
#5584=DIRECTION ( 'NONE',  ( -0.000000000000000000, 0.000000000000000000, -1.000000000000000000 ) ) ;
#5594=CIRCLE ( 'NONE', #14204, 0.7892041907098262810 ) ;
#5604=AXIS2_PLACEMENT_3D ( 'NONE', #11264, #1876, #722 ) ;
#5606=AXIS2_PLACEMENT_3D ( 'NONE', #10230, #983, #5622 ) ;
#5607=ORIENTED_EDGE ( 'NONE', *, *, #7153, .T. ) ;
#5611=EDGE_CURVE ( 'NONE', #9619, #12270, #7057, .T. ) ;
#5619=DIRECTION ( 'NONE',  ( 0.4331347858759544978, 0.9013291614411413910, 0.000000000000000000 ) ) ;
#5620=AXIS2_PLACEMENT_3D ( 'NONE', #3081, #9003, #5394 ) ;
#5622=DIRECTION ( 'NONE',  ( 0.8746197071345563900, -0.4848096202550675193, 0.000000000000000000 ) ) ;
#5624=DIRECTION ( 'NONE',  ( 0.8746197071345569451, -0.4848096202550666312, 0.000000000000000000 ) ) ;
#5625=ORIENTED_EDGE ( 'NONE', *, *, #11025, .F. ) ;
#5627=DIRECTION ( 'NONE',  ( 0.5640065580417802371, -0.8257703085518780517, 0.000000000000000000 ) ) ;
#5629=CARTESIAN_POINT ( 'NONE',  ( 69.46410738159350728, -2.362204130743390085, 75.71883071479155092 ) ) ;
#5633=ORIENTED_EDGE ( 'NONE', *, *, #2217, .F. ) ;
#5647=CIRCLE ( 'NONE', #14718, 1.000000000000000888 ) ;
#5649=CARTESIAN_POINT ( 'NONE',  ( 54.86190032082818391, 1.721056973166403603, 48.51982618741349285 ) ) ;
#5672=ORIENTED_EDGE ( 'NONE', *, *, #3765, .T. ) ;
#5681=CARTESIAN_POINT ( 'NONE',  ( 53.41380296247595538, -0.1096349785133995947, 62.84860122826521689 ) ) ;
#5683=EDGE_CURVE ( 'NONE', #6506, #5691, #10680, .T. ) ;
#5684=ORIENTED_EDGE ( 'NONE', *, *, #2459, .T. ) ;
#5689=DIRECTION ( 'NONE',  ( 0.3020115420618306734, -0.1674077314120155646, 0.9384901064608606180 ) ) ;
#5690=( BOUNDED_SURFACE ( )  B_SPLINE_SURFACE ( 3, 2, ( 
 ( #12395, #7346, #7706 ),
 ( #6207, #1420, #13621 ),
 ( #13473, #7779, #4965 ),
 ( #4299, #14620, #12319 ),
 ( #4152, #11163, #11232 ),
 ( #12035, #3802, #8506 ),
 ( #2934, #7626, #5316 ),
 ( #1498, #3012, #10088 ),
 ( #14774, #8930, #10893 ),
 ( #12469, #539, #2316 ),
 ( #3469, #5871, #9086 ),
 ( #7, #1077, #11695 ),
 ( #6930, #11453, #13932 ),
 ( #3232, #10237, #11620 ) ),
 .UNSPECIFIED., .F., .F., .F. ) 
 B_SPLINE_SURFACE_WITH_KNOTS ( ( 4, 2, 2, 2, 2, 2, 4 ),
 ( 3, 3 ),
 ( 0.001417163504557058824, 0.002234205688869395946, 0.002642726781025564291, 0.003051247873181732635, 0.003459768965337900980, 0.003868290057494069758, 0.004685332241806406881 ),
 ( 0.000000000000000000, 1.000000000000000000 ),
 .UNSPECIFIED. ) 
 GEOMETRIC_REPRESENTATION_ITEM ( )  RATIONAL_B_SPLINE_SURFACE ( (
 ( 1.000000000000000000, 0.7071067811865471286, 1.000000000000000000),
 ( 1.000000000000000000, 0.7218508617828192087, 1.000000000000000000),
 ( 1.000000000000000000, 0.7387008909040627680, 1.000000000000000000),
 ( 1.000000000000000000, 0.7647615808954046912, 1.000000000000000000),
 ( 1.000000000000000000, 0.7734065576773767603, 1.000000000000000000),
 ( 1.000000000000000000, 0.7903558204260539011, 1.000000000000000000),
 ( 1.000000000000000000, 0.7987454157985085512, 1.000000000000000000),
 ( 1.000000000000000000, 0.8144265709899989325, 1.000000000000000000),
 ( 1.000000000000000000, 0.8216999247152600994, 1.000000000000000000),
 ( 1.000000000000000000, 0.8348485599607926577, 1.000000000000000000),
 ( 1.000000000000000000, 0.8407795038256219433, 1.000000000000000000),
 ( 1.000000000000000000, 0.8552130772092386701, 1.000000000000000000),
 ( 1.000000000000000000, 0.8606507091652410013, 1.000000000000000000),
 ( 1.000000000000000000, 0.8606282562001379421, 1.000000000000000000) ) ) 
 REPRESENTATION_ITEM ( '' )  SURFACE ( )  );
#5691=VERTEX_POINT ( 'NONE', #14220 ) ;
#5694=ORIENTED_EDGE ( 'NONE', *, *, #5504, .F. ) ;
#5705=TOROIDAL_SURFACE ( 'NONE', #14045, 3.999999999999996447, 1.000000000000000000 ) ;
#5712=DIRECTION ( 'NONE',  ( 0.8746197071345569451, -0.4848096202550666312, 0.000000000000000000 ) ) ;
#5720=CARTESIAN_POINT ( 'NONE',  ( 58.00000000000000711, -2.249290599286309256, 39.50000000000012790 ) ) ;
#5721=CARTESIAN_POINT ( 'NONE',  ( 64.11356537587559501, -11.94785244090458498, 75.19766410831374515 ) ) ;
#5728=EDGE_LOOP ( 'NONE', ( #3902, #10424, #11858, #1298 ) ) ;
#5730=AXIS2_PLACEMENT_3D ( 'NONE', #14763, #3005, #2209 ) ;
#5736=AXIS2_PLACEMENT_3D ( 'NONE', #9496, #6190, #14263 ) ;
#5738=DIRECTION ( 'NONE',  ( 0.8746197071345569451, -0.4848096202550666312, 0.000000000000000000 ) ) ;
#5745=AXIS2_PLACEMENT_3D ( 'NONE', #10148, #4440, #1902 ) ;
#5752=CARTESIAN_POINT ( 'NONE',  ( 60.34603303165619792, -7.282908750500069139, 48.51982618741349285 ) ) ;
#5756=DIRECTION ( 'NONE',  ( 0.8746197071345569451, -0.4848096202550666312, 0.000000000000000000 ) ) ;
#5763=ADVANCED_FACE ( 'NONE', ( #2743 ), #2884, .T. ) ;
#5769=ORIENTED_EDGE ( 'NONE', *, *, #10543, .T. ) ;
#5773=DIRECTION ( 'NONE',  ( 0.000000000000000000, 0.000000000000000000, 1.000000000000000000 ) ) ;
#5780=ORIENTED_EDGE ( 'NONE', *, *, #4897, .T. ) ;
#5787=CARTESIAN_POINT ( 'NONE',  ( 58.00000000000000711, -2.249290599286311032, 38.50000000000012790 ) ) ;
#5796=CARTESIAN_POINT ( 'NONE',  ( 54.21883389619742388, -5.612936290787406968, 48.51982618741349285 ) ) ;
#5806=DIRECTION ( 'NONE',  ( -0.2475627213817241101, 0.9688718692283695422, 0.000000000000000000 ) ) ;
#5817=CARTESIAN_POINT ( 'NONE',  ( 62.14930354033766946, 1.441842398587373619, 54.56811043785582882 ) ) ;
#5835=DIRECTION ( 'NONE',  ( -0.8208219420614785156, 0.4549890321264269399, 0.3453061251629920836 ) ) ;
#5849=ORIENTED_EDGE ( 'NONE', *, *, #13360, .F. ) ;
#5854=PRODUCT_DEFINITION_FORMATION_WITH_SPECIFIED_SOURCE ( 'ANY', '', #6577, .NOT_KNOWN. ) ;
#5855=ORIENTED_EDGE ( 'NONE', *, *, #6742, .T. ) ;
#5859=EDGE_CURVE ( 'NONE', #11327, #8779, #4987, .T. ) ;
#5860=CIRCLE ( 'NONE', #10519, 0.7892041907098275022 ) ;
#5866=CARTESIAN_POINT ( 'NONE',  ( 70.01073691755573236, -3.266485040426043263, 72.83188032674053147 ) ) ;
#5871=CARTESIAN_POINT ( 'NONE',  ( 64.77045472790173619, -11.51823327494775384, 72.60588509441274141 ) ) ;
#5874=CIRCLE ( 'NONE', #3642, 0.9999999999999957812 ) ;
#5876=CARTESIAN_POINT ( 'NONE',  ( 69.36577990805442084, -3.791597611828531278, 72.16308916778781679 ) ) ;
#5888=CARTESIAN_POINT ( 'NONE',  ( 119.4687373431154782, -36.32196809074999777, 57.22220354671986087 ) ) ;
#5891=ORIENTED_EDGE ( 'NONE', *, *, #6605, .F. ) ;
#5892=DIRECTION ( 'NONE',  ( 0.000000000000000000, 0.000000000000000000, 1.000000000000000000 ) ) ;
#5896=LINE ( 'NONE', #40, #7060 ) ;
#5904=CARTESIAN_POINT ( 'NONE',  ( 69.97972559857382180, -3.172990593254279457, 73.19766410831374515 ) ) ;
#5908=ORIENTED_EDGE ( 'NONE', *, *, #8333, .F. ) ;
#5909=DIRECTION ( 'NONE',  ( -0.8746197071345569451, 0.4848096202550666312, 0.000000000000000000 ) ) ;
#5914=CARTESIAN_POINT ( 'NONE',  ( 64.11356537587560922, -11.94785244090458853, 75.19766410831373094 ) ) ;
#5915=CARTESIAN_POINT ( 'NONE',  ( 58.00000000000000711, -2.249290599286309256, 81.40005259842790508 ) ) ;
#5920=VECTOR ( 'NONE', #5440, 1000.000000000000000 ) ;
#5924=VERTEX_POINT ( 'NONE', #3645 ) ;
#5928=DIRECTION ( 'NONE',  ( 0.000000000000000000, 0.000000000000000000, 1.000000000000000000 ) ) ;
#5930=ORIENTED_EDGE ( 'NONE', *, *, #14122, .T. ) ;
#5932=CARTESIAN_POINT ( 'NONE',  ( 53.19261734817368392, 0.4154851184807626940, 87.40005259842790508 ) ) ;
#5936=DIRECTION ( 'NONE',  ( 0.9628490124547428586, -0.2700403288676087032, 0.000000000000000000 ) ) ;
#5939=AXIS2_PLACEMENT_3D ( 'NONE', #9440, #10815, #4966 ) ;
#5940=CARTESIAN_POINT ( 'NONE',  ( 67.15257324181105503, -7.322644791425995336, 82.40005259842790508 ) ) ;
#5942=EDGE_CURVE ( 'NONE', #13455, #12270, #14570, .T. ) ;
#5944=ORIENTED_EDGE ( 'NONE', *, *, #4515, .F. ) ;
#5946=CARTESIAN_POINT ( 'NONE',  ( 70.17101333207268965, -3.861229032418910467, 72.32404137764891061 ) ) ;
#5947=CIRCLE ( 'NONE', #11827, 4.496540510819673209 ) ;
#5954=AXIS2_PLACEMENT_3D ( 'NONE', #6032, #26, #14185 ) ;
#5966=EDGE_CURVE ( 'NONE', #6435, #14286, #4301, .T. ) ;
#5969=ORIENTED_EDGE ( 'NONE', *, *, #13140, .F. ) ;
#5974=CARTESIAN_POINT ( 'NONE',  ( 87.44800360084714441, -24.28935588223203723, -34.74844256990415658 ) ) ;
#5975=AXIS2_PLACEMENT_3D ( 'NONE', #14120, #39, #8502 ) ;
#5980=DIRECTION ( 'NONE',  ( 0.000000000000000000, 0.000000000000000000, 1.000000000000000000 ) ) ;
#5982=FACE_OUTER_BOUND ( 'NONE', #13349, .T. ) ;
#5983=CIRCLE ( 'NONE', #11867, 0.7892041907098262810 ) ;
#5985=ORIENTED_EDGE ( 'NONE', *, *, #8091, .T. ) ;
#5994=CARTESIAN_POINT ( 'NONE',  ( 64.61411691182246386, -11.63232581036083246, 75.19766410831375936 ) ) ;
#6013=LINE ( 'NONE', #12934, #2624 ) ;
#6014=PLANE ( 'NONE',  #14586 ) ;
#6022=EDGE_LOOP ( 'NONE', ( #11568, #4224, #5607, #12440 ) ) ;
#6025=DIRECTION ( 'NONE',  ( -0.000000000000000000, 0.000000000000000000, -1.000000000000000000 ) ) ;
#6027=ORIENTED_EDGE ( 'NONE', *, *, #8670, .T. ) ;
#6032=CARTESIAN_POINT ( 'NONE',  ( 76.14589960879429498, -7.734310727912404815, 75.19766410831374515 ) ) ;
#6039=DIRECTION ( 'NONE',  ( 0.8746197071345563900, -0.4848096202550675193, 0.000000000000000000 ) ) ;
#6049=CARTESIAN_POINT ( 'NONE',  ( 65.71319926014255941, -10.73129157630437547, 71.19766410831374515 ) ) ;
#6059=CARTESIAN_POINT ( 'NONE',  ( 66.10056138690445948, -11.60665394596473021, 76.17249640597626126 ) ) ;
#6061=CIRCLE ( 'NONE', #6780, 0.7892041907098262810 ) ;
#6065=EDGE_CURVE ( 'NONE', #7654, #6506, #5483, .T. ) ;
#6067=CARTESIAN_POINT ( 'NONE',  ( 59.12196317473677709, -7.688259372168277928, 54.56811043785583593 ) ) ;
#6072=TOROIDAL_SURFACE ( 'NONE', #5324, 7.924024642120688355, 1.000000000000000000 ) ;
#6076=EDGE_LOOP ( 'NONE', ( #2438, #2477, #14369, #9600 ) ) ;
#6081=CARTESIAN_POINT ( 'NONE',  ( 69.28051765693513175, -4.295678830383772961, 71.19766410831374515 ) ) ;
#6083=ORIENTED_EDGE ( 'NONE', *, *, #11676, .T. ) ;
#6086=DIRECTION ( 'NONE',  ( 0.000000000000000000, 0.000000000000000000, 1.000000000000000000 ) ) ;
#6090=DIRECTION ( 'NONE',  ( 0.000000000000000000, 0.000000000000000000, 1.000000000000000000 ) ) ;
#6098=CIRCLE ( 'NONE', #7316, 0.7892041907098262810 ) ;
#6106=ADVANCED_FACE ( 'NONE', ( #12397 ), #8910, .T. ) ;
#6112=CARTESIAN_POINT ( 'NONE',  ( 53.04398595309534414, -1.224959495890951100, 62.84860122826521689 ) ) ;
#6115=AXIS2_PLACEMENT_3D ( 'NONE', #6994, #978, #4684 ) ;
#6116=CARTESIAN_POINT ( 'NONE',  ( 56.28732689558331259, 3.089731932287650640, 62.84860122826521689 ) ) ;
#6117=VERTEX_POINT ( 'NONE', #11235 ) ;
#6119=LINE ( 'NONE', #14198, #6213 ) ;
#6124=CARTESIAN_POINT ( 'NONE',  ( 76.44791115085612887, -7.901718459324428068, 76.13615421477460643 ) ) ;
#6127=CARTESIAN_POINT ( 'NONE',  ( 70.08269333764698672, -3.500995332129508864, 75.85600374239184873 ) ) ;
#6131=ORIENTED_EDGE ( 'NONE', *, *, #10943, .T. ) ;
#6138=ORIENTED_EDGE ( 'NONE', *, *, #15155, .F. ) ;
#6139=CARTESIAN_POINT ( 'NONE',  ( 64.66512137289342377, -11.59558090713824541, 75.55235509932406046 ) ) ;
#6141=CARTESIAN_POINT ( 'NONE',  ( 58.00000000000000711, -2.249290599286309256, 47.51982618741348574 ) ) ;
#6145=VERTEX_POINT ( 'NONE', #12706 ) ;
#6153=ORIENTED_EDGE ( 'NONE', *, *, #3318, .F. ) ;
#6154=EDGE_CURVE ( 'NONE', #3899, #5063, #3764, .T. ) ;
#6157=DIRECTION ( 'NONE',  ( -0.8746197071345569451, 0.4848096202550666312, 0.000000000000000000 ) ) ;
#6163=ORIENTED_EDGE ( 'NONE', *, *, #2016, .T. ) ;
#6165=DIRECTION ( 'NONE',  ( -0.8746197071345572782, 0.4848096202550659650, -0.000000000000000000 ) ) ;
#6169=CARTESIAN_POINT ( 'NONE',  ( 66.38598137497019991, -11.47113225237460199, 71.19766410831374515 ) ) ;
#6176=VERTEX_POINT ( 'NONE', #15014 ) ;
#6177=ADVANCED_FACE ( 'NONE', ( #4461 ), #9171, .T. ) ;
#6181=VERTEX_POINT ( 'NONE', #3391 ) ;
#6182=SHAPE_DEFINITION_REPRESENTATION ( #14687, #11972 ) ;
#6189=DIRECTION ( 'NONE',  ( -0.8746197071345569451, 0.4848096202550666312, 0.000000000000000000 ) ) ;
#6190=DIRECTION ( 'NONE',  ( -0.8208219420614839557, 0.4549890321264298820, 0.3453061251629756523 ) ) ;
#6195=EDGE_CURVE ( 'NONE', #11917, #604, #3279, .T. ) ;
#6196=AXIS2_PLACEMENT_3D ( 'NONE', #10419, #2482, #4715 ) ;
#6198=ADVANCED_FACE ( 'NONE', ( #2235 ), #6931, .F. ) ;
#6203=CARTESIAN_POINT ( 'NONE',  ( 69.46467306388282736, -2.354974971177655085, 75.74364963835485298 ) ) ;
#6207=CARTESIAN_POINT ( 'NONE',  ( 65.52631879429515038, -10.90123334768769858, 71.19766412131004074 ) ) ;
#6212=CYLINDRICAL_SURFACE ( 'NONE', #11794, 0.7892041907098262810 ) ;
#6213=VECTOR ( 'NONE', #3655, 1000.000000000000000 ) ;
#6215=CARTESIAN_POINT ( 'NONE',  ( 66.92402464212069901, -2.249290599286308368, 47.51982618741348574 ) ) ;
#6216=AXIS2_PLACEMENT_3D ( 'NONE', #13255, #7548, #536 ) ;
#6229=VECTOR ( 'NONE', #12321, 1000.000000000000000 ) ;
#6230=EDGE_CURVE ( 'NONE', #7295, #12140, #9682, .T. ) ;
#6233=CARTESIAN_POINT ( 'NONE',  ( 71.80003071982790175, -14.47218880931180962, 72.19766410831374515 ) ) ;
#6241=CARTESIAN_POINT ( 'NONE',  ( 65.80512781895316721, -6.575743597179691591, 82.40005259842790508 ) ) ;
#6250=DIRECTION ( 'NONE',  ( 0.000000000000000000, -1.000000000000000000, 0.000000000000000000 ) ) ;
#6253=CARTESIAN_POINT ( 'NONE',  ( 65.13162939602317181, -11.91918766459985157, 73.19766410831374515 ) ) ;
#6254=ORIENTED_EDGE ( 'NONE', *, *, #5859, .F. ) ;
#6269=DIRECTION ( 'NONE',  ( 0.8208219420614785156, -0.4549890321264269399, -0.3453061251629920836 ) ) ;
#6270=CARTESIAN_POINT ( 'NONE',  ( 69.46454297106443221, -2.294433322023685662, 75.19766410831374515 ) ) ;
#6271=CARTESIAN_POINT ( 'NONE',  ( 64.11356537587559501, -11.94785244090458498, 73.19766410831374515 ) ) ;
#6281=ORIENTED_EDGE ( 'NONE', *, *, #10684, .F. ) ;
#6287=VERTEX_POINT ( 'NONE', #1233 ) ;
#6300=CARTESIAN_POINT ( 'NONE',  ( 72.12120841366726154, -14.65022051213588128, 75.25917400185288386 ) ) ;
#6302=ORIENTED_EDGE ( 'NONE', *, *, #9100, .F. ) ;
#6306=AXIS2_PLACEMENT_3D ( 'NONE', #8255, #12951, #100 ) ;
#6308=CYLINDRICAL_SURFACE ( 'NONE', #11559, 0.7892041907098261699 ) ;
#6311=ORIENTED_EDGE ( 'NONE', *, *, #6369, .T. ) ;
#6312=CARTESIAN_POINT ( 'NONE',  ( 65.18587381434291217, -11.90669967090665793, 72.89354184684002291 ) ) ;
#6315=AXIS2_PLACEMENT_3D ( 'NONE', #4082, #8567, #11096 ) ;
#6321=CIRCLE ( 'NONE', #8296, 8.924024642120691908 ) ;
#6328=CIRCLE ( 'NONE', #644, 8.924024642120691908 ) ;
#6342=AXIS2_PLACEMENT_3D ( 'NONE', #8554, #9237, #6610 ) ;
#6346=CARTESIAN_POINT ( 'NONE',  ( 62.80738265182633739, -4.914066317053381816, 86.40005259842790508 ) ) ;
#6354=CARTESIAN_POINT ( 'NONE',  ( 53.34060950309435611, 1.272953934520814290, 62.84860122826521689 ) ) ;
#6355=EDGE_LOOP ( 'NONE', ( #515, #12133, #6737 ) ) ;
#6362=CARTESIAN_POINT ( 'NONE',  ( 54.30726695196912601, -6.397170215889376621, 48.51982618741349285 ) ) ;
#6369=EDGE_CURVE ( 'NONE', #14121, #5503, #2295, .T. ) ;
#6380=DIRECTION ( 'NONE',  ( -0.8746197071345570562, 0.4848096202550665756, 0.000000000000000000 ) ) ;
#6387=AXIS2_PLACEMENT_3D ( 'NONE', #7110, #4879, #1255 ) ;
#6390=EDGE_CURVE ( 'NONE', #12128, #14607, #2837, .T. ) ;
#6391=CARTESIAN_POINT ( 'NONE',  ( 58.00000000000000711, -2.249290599286309256, 72.19766410831374515 ) ) ;
#6392=FACE_OUTER_BOUND ( 'NONE', #10427, .T. ) ;
#6404=CARTESIAN_POINT ( 'NONE',  ( 62.80738265182633739, -4.914066317053381816, 82.40005259842790508 ) ) ;
#6405=EDGE_LOOP ( 'NONE', ( #7562, #1649, #13675, #1595 ) ) ;
#6409=EDGE_CURVE ( 'NONE', #9304, #11686, #5495, .T. ) ;
#6410=VECTOR ( 'NONE', #7376, 999.9999999999998863 ) ;
#6412=CARTESIAN_POINT ( 'NONE',  ( 58.00000000000000711, -2.249290599286309256, 48.51982618741349285 ) ) ;
#6413=CARTESIAN_POINT ( 'NONE',  ( 71.94624495291445498, -14.55323668216481536, 72.13615421477459222 ) ) ;
#6416=DIRECTION ( 'NONE',  ( 0.8746197071345569451, -0.4848096202550666312, 0.000000000000000000 ) ) ;
#6420=ORIENTED_EDGE ( 'NONE', *, *, #10684, .T. ) ;
#6421=CIRCLE ( 'NONE', #15030, 0.7892041907098250597 ) ;
#6435=VERTEX_POINT ( 'NONE', #5456 ) ;
#6437=ORIENTED_EDGE ( 'NONE', *, *, #1419, .F. ) ;
#6438=CARTESIAN_POINT ( 'NONE',  ( 66.38598137497019991, -11.47113225237460910, 72.19766410831374515 ) ) ;
#6441=DIRECTION ( 'NONE',  ( 0.000000000000000000, 0.000000000000000000, 1.000000000000000000 ) ) ;
#6445=ORIENTED_EDGE ( 'NONE', *, *, #4035, .T. ) ;
#6451=DIRECTION ( 'NONE',  ( -0.000000000000000000, 0.000000000000000000, -1.000000000000000000 ) ) ;
#6457=ORIENTED_EDGE ( 'NONE', *, *, #311, .F. ) ;
#6461=ORIENTED_EDGE ( 'NONE', *, *, #1829, .T. ) ;
#6464=AXIS2_PLACEMENT_3D ( 'NONE', #12196, #12132, #363 ) ;
#6465=DIRECTION ( 'NONE',  ( -0.000000000000000000, 0.000000000000000000, -1.000000000000000000 ) ) ;
#6467=DIRECTION ( 'NONE',  ( 0.8746197071345571672, -0.4848096202550660205, 0.000000000000000000 ) ) ;
#6468=CARTESIAN_POINT ( 'NONE',  ( 58.00000000000000711, -2.249290599286309256, 71.19766410831374515 ) ) ;
#6470=ADVANCED_FACE ( 'NONE', ( #14755 ), #13528, .F. ) ;
#6473=CARTESIAN_POINT ( 'NONE',  ( 63.55116547662792215, -2.088839582009629936, 54.56811043785582882 ) ) ;
#6474=DIRECTION ( 'NONE',  ( -0.000000000000000000, 0.000000000000000000, -1.000000000000000000 ) ) ;
#6475=AXIS2_PLACEMENT_3D ( 'NONE', #9400, #3470, #2317 ) ;
#6488=CYLINDRICAL_SURFACE ( 'NONE', #5147, 0.7892041907098262810 ) ;
#6506=VERTEX_POINT ( 'NONE', #11215 ) ;
#6514=LINE ( 'NONE', #9143, #818 ) ;
#6522=VERTEX_POINT ( 'NONE', #3070 ) ;
#6534=CARTESIAN_POINT ( 'NONE',  ( 53.19261734817368392, 0.4154851184807644149, 86.40005259842790508 ) ) ;
#6537=DIRECTION ( 'NONE',  ( -1.000000000000000000, 0.000000000000000000, 0.000000000000000000 ) ) ;
#6542=AXIS2_PLACEMENT_3D ( 'NONE', #9310, #3686, #232 ) ;
#6544=CARTESIAN_POINT ( 'NONE',  ( 53.34060950309435611, 1.272953934520814734, 60.61639468829817190 ) ) ;
#6546=( NAMED_UNIT ( * ) PLANE_ANGLE_UNIT ( ) SI_UNIT ( $, .RADIAN. ) );
#6553=CIRCLE ( 'NONE', #12200, 2.000000000000001776 ) ;
#6554=CARTESIAN_POINT ( 'NONE',  ( 72.26742264675378635, -14.73126838498887281, 75.19766410831374515 ) ) ;
#6555=AXIS2_PLACEMENT_3D ( 'NONE', #2718, #11097, #7419 ) ;
#6563=VERTEX_POINT ( 'NONE', #13760 ) ;
#6571=CARTESIAN_POINT ( 'NONE',  ( 76.61154307727187529, -6.849067049365817006, 73.07464432123545350 ) ) ;
#6573=AXIS2_PLACEMENT_3D ( 'NONE', #2473, #9640, #1547 ) ;
#6574=CARTESIAN_POINT ( 'NONE',  ( 71.64423341085262109, -14.38582895075278500, 73.19766410831374515 ) ) ;
#6576=ADVANCED_FACE ( 'NONE', ( #11435 ), #1129, .T. ) ;
#6577=PRODUCT ( 'Locking Handle', 'Locking Handle', '', ( #9648 ) ) ;
#6578=VECTOR ( 'NONE', #9731, 1000.000000000000000 ) ;
#6587=ORIENTED_EDGE ( 'NONE', *, *, #7287, .F. ) ;
#6588=DIRECTION ( 'NONE',  ( 0.8746197071345570562, -0.4848096202550662981, 0.000000000000000000 ) ) ;
#6591=CYLINDRICAL_SURFACE ( 'NONE', #8762, 0.7892041907098262810 ) ;
#6596=VERTEX_POINT ( 'NONE', #11600 ) ;
#6602=CARTESIAN_POINT ( 'NONE',  ( 76.00751999314820750, -6.514251586541772276, 71.19766410831374515 ) ) ;
#6603=ORIENTED_EDGE ( 'NONE', *, *, #74, .F. ) ;
#6605=EDGE_CURVE ( 'NONE', #11544, #1585, #10011, .T. ) ;
#6606=ORIENTED_EDGE ( 'NONE', *, *, #5328, .T. ) ;
#6610=DIRECTION ( 'NONE',  ( -0.5348440123420857839, -0.8449508165933795611, 0.000000000000000000 ) ) ;
#6612=CIRCLE ( 'NONE', #7595, 0.7892041907098298337 ) ;
#6616=LINE ( 'NONE', #6473, #932 ) ;
#6620=DIRECTION ( 'NONE',  ( -0.000000000000000000, 0.000000000000000000, -1.000000000000000000 ) ) ;
#6622=ADVANCED_FACE ( 'NONE', ( #899 ), #2140, .T. ) ;
#6624=AXIS2_PLACEMENT_3D ( 'NONE', #14195, #5892, #4645 ) ;
#6629=CARTESIAN_POINT ( 'NONE',  ( 53.54504563787001814, -4.650271872399136086, 48.51982618741349285 ) ) ;
#6635=CARTESIAN_POINT ( 'NONE',  ( 60.45350693790843621, 2.176953084486059176, 60.61639468829817190 ) ) ;
#6638=EDGE_CURVE ( 'NONE', #1585, #11588, #8462, .T. ) ;
#6645=EDGE_LOOP ( 'NONE', ( #7715, #3936, #4430, #6027 ) ) ;
#6646=DIRECTION ( 'NONE',  ( 0.8746197071345569451, -0.4848096202550666312, 0.000000000000000000 ) ) ;
#6648=FACE_OUTER_BOUND ( 'NONE', #8315, .T. ) ;
#6651=CARTESIAN_POINT ( 'NONE',  ( 65.71319926014255941, -10.73129157630437547, 77.19766410831374515 ) ) ;
#6659=CARTESIAN_POINT ( 'NONE',  ( 116.7426776997783406, -40.52765889501078078, 56.28371344025899248 ) ) ;
#6677=ORIENTED_EDGE ( 'NONE', *, *, #4991, .F. ) ;
#6687=EDGE_CURVE ( 'NONE', #6563, #1582, #11904, .T. ) ;
#6690=VECTOR ( 'NONE', #3611, 1000.000000000000000 ) ;
#6692=EDGE_LOOP ( 'NONE', ( #12547, #12948, #6420, #9012, #3778 ) ) ;
#6695=CARTESIAN_POINT ( 'NONE',  ( 69.46039030023230509, -2.569771090503329525, 76.19917534039397822 ) ) ;
#6705=DIRECTION ( 'NONE',  ( 0.000000000000000000, 0.000000000000000000, 1.000000000000000000 ) ) ;
#6707=ORIENTED_EDGE ( 'NONE', *, *, #14855, .F. ) ;
#6710=CARTESIAN_POINT ( 'NONE',  ( 52.25109540565180311, -2.012892184189034595, 60.61639468829817190 ) ) ;
#6718=EDGE_LOOP ( 'NONE', ( #7372, #14107, #1594, #8452 ) ) ;
#6720=EDGE_LOOP ( 'NONE', ( #243, #14726, #3107, #2212 ) ) ;
#6724=ORIENTED_EDGE ( 'NONE', *, *, #10598, .F. ) ;
#6725=DIRECTION ( 'NONE',  ( 0.000000000000000000, 0.000000000000000000, 1.000000000000000000 ) ) ;
#6737=ORIENTED_EDGE ( 'NONE', *, *, #11676, .F. ) ;
#6742=EDGE_CURVE ( 'NONE', #6145, #12282, #9784, .T. ) ;
#6743=FACE_OUTER_BOUND ( 'NONE', #7374, .T. ) ;
#6747=FACE_OUTER_BOUND ( 'NONE', #8680, .T. ) ;
#6756=ORIENTED_EDGE ( 'NONE', *, *, #9001, .T. ) ;
#6757=PLANE ( 'NONE',  #2014 ) ;
#6764=CIRCLE ( 'NONE', #149, 0.7892041907098241715 ) ;
#6767=CARTESIAN_POINT ( 'NONE',  ( 69.40538204389208943, -3.419623080944494742, 76.98915142890231778 ) ) ;
#6768=ADVANCED_FACE ( 'NONE', ( #10834 ), #1523, .T. ) ;
#6777=CARTESIAN_POINT ( 'NONE',  ( 61.93276294469178822, -4.429256696798314685, 87.40005259842790508 ) ) ;
#6780=AXIS2_PLACEMENT_3D ( 'NONE', #7016, #10636, #1240 ) ;
#6784=PLANE ( 'NONE',  #2606 ) ;
#6793=ORIENTED_EDGE ( 'NONE', *, *, #11222, .F. ) ;
#6803=DIRECTION ( 'NONE',  ( 0.6293203910575899673, 0.7771459614506929237, 0.000000000000000000 ) ) ;
#6806=DIRECTION ( 'NONE',  ( -0.000000000000000000, 0.000000000000000000, -1.000000000000000000 ) ) ;
#6810=CARTESIAN_POINT ( 'NONE',  ( 52.94134894379979528, -2.395505968190773327, 60.61639468829817190 ) ) ;
#6811=AXIS2_PLACEMENT_3D ( 'NONE', #12586, #2195, #2038 ) ;
#6812=FACE_OUTER_BOUND ( 'NONE', #3071, .T. ) ;
#6813=ORIENTED_EDGE ( 'NONE', *, *, #1123, .T. ) ;
#6823=AXIS2_PLACEMENT_3D ( 'NONE', #8211, #5980, #1267 ) ;
#6824=DIRECTION ( 'NONE',  ( -0.000000000000000000, 0.000000000000000000, -1.000000000000000000 ) ) ;
#6825=CIRCLE ( 'NONE', #13711, 0.7892041907098288345 ) ;
#6832=ADVANCED_FACE ( 'NONE', ( #1815 ), #13586, .T. ) ;
#6837=LINE ( 'NONE', #8991, #1284 ) ;
#6838=AXIS2_PLACEMENT_3D ( 'NONE', #4225, #9946, #6537 ) ;
#6844=DIRECTION ( 'NONE',  ( 1.000000000000000000, 0.000000000000000000, 0.000000000000000000 ) ) ;
#6846=CARTESIAN_POINT ( 'NONE',  ( 76.00751999314820750, -6.514251586541772276, 71.19766410831374515 ) ) ;
#6855=DIRECTION ( 'NONE',  ( 1.000000000000000000, 0.000000000000000000, 0.000000000000000000 ) ) ;
#6858=AXIS2_PLACEMENT_3D ( 'NONE', #6635, #11250, #702 ) ;
#6870=DIRECTION ( 'NONE',  ( 0.000000000000000000, 0.000000000000000000, 1.000000000000000000 ) ) ;
#6873=ORIENTED_EDGE ( 'NONE', *, *, #3343, .T. ) ;
#6883=CIRCLE ( 'NONE', #260, 11.46463184759104870 ) ;
#6894=VERTEX_POINT ( 'NONE', #8731 ) ;
#6907=CARTESIAN_POINT ( 'NONE',  ( 48.84742675818896629, 2.824063592853376381, 82.40005259842790508 ) ) ;
#6909=DIRECTION ( 'NONE',  ( -0.8208219420614786266, 0.4549890321264269399, 0.3453061251629919171 ) ) ;
#6912=VERTEX_POINT ( 'NONE', #6362 ) ;
#6930=CARTESIAN_POINT ( 'NONE',  ( 64.11356537427461433, -11.94785244191377949, 72.92170383108769727 ) ) ;
#6931=PLANE ( 'NONE',  #6475 ) ;
#6934=MECHANICAL_DESIGN_GEOMETRIC_PRESENTATION_REPRESENTATION('',(#12580),#12335);
#6939=DIRECTION ( 'NONE',  ( -0.8746197071345569451, 0.4848096202550666312, 0.000000000000000000 ) ) ;
#6955=DIRECTION ( 'NONE',  ( 0.000000000000000000, 0.000000000000000000, 1.000000000000000000 ) ) ;
#6968=FACE_OUTER_BOUND ( 'NONE', #13690, .T. ) ;
#6972=CYLINDRICAL_SURFACE ( 'NONE', #4109, 0.7892041907098262810 ) ;
#6973=AXIS2_PLACEMENT_3D ( 'NONE', #8069, #6909, #5689 ) ;
#6978=ORIENTED_EDGE ( 'NONE', *, *, #10774, .F. ) ;
#6983=CARTESIAN_POINT ( 'NONE',  ( 64.69561927709757754, -11.57345611214739733, 75.63685169989432211 ) ) ;
#6992=ORIENTED_EDGE ( 'NONE', *, *, #14702, .T. ) ;
#6994=CARTESIAN_POINT ( 'NONE',  ( 118.5627027169299765, -35.81974489651393156, 54.40673322733726280 ) ) ;
#6997=ORIENTED_EDGE ( 'NONE', *, *, #8732, .T. ) ;
#7001=CYLINDRICAL_SURFACE ( 'NONE', #3256, 0.7892041907098262810 ) ;
#7004=CARTESIAN_POINT ( 'NONE',  ( 76.30953153521004140, -6.681659317953794641, 72.13615421477459222 ) ) ;
#7014=ADVANCED_FACE ( 'NONE', ( #3432 ), #6972, .T. ) ;
#7016=CARTESIAN_POINT ( 'NONE',  ( 59.59091026602544616, -7.053490217115945704, 60.61639468829817190 ) ) ;
#7025=DIRECTION ( 'NONE',  ( -0.000000000000000000, 0.000000000000000000, -1.000000000000000000 ) ) ;
#7030=VECTOR ( 'NONE', #7565, 1000.000000000000000 ) ;
#7046=DIRECTION ( 'NONE',  ( 0.000000000000000000, 0.000000000000000000, 1.000000000000000000 ) ) ;
#7052=AXIS2_PLACEMENT_3D ( 'NONE', #4901, #14219, #12993 ) ;
#7053=ORIENTED_EDGE ( 'NONE', *, *, #196, .F. ) ;
#7057=LINE ( 'NONE', #1281, #2770 ) ;
#7060=VECTOR ( 'NONE', #3422, 1000.000000000000000 ) ;
#7062=ORIENTED_EDGE ( 'NONE', *, *, #10491, .T. ) ;
#7065=DIRECTION ( 'NONE',  ( 0.000000000000000000, 0.000000000000000000, 1.000000000000000000 ) ) ;
#7078=AXIS2_PLACEMENT_3D ( 'NONE', #5787, #9243, #6844 ) ;
#7084=ADVANCED_FACE ( 'NONE', ( #6812 ), #2645, .T. ) ;
#7094=CARTESIAN_POINT ( 'NONE',  ( 69.32915027133518038, -4.025971040916268784, 72.13752247958439057 ) ) ;
#7095=ORIENTED_EDGE ( 'NONE', *, *, #5180, .F. ) ;
#7098=ORIENTED_EDGE ( 'NONE', *, *, #10420, .F. ) ;
#7100=DIRECTION ( 'NONE',  ( -0.000000000000000000, 0.000000000000000000, -1.000000000000000000 ) ) ;
#7101=ORIENTED_EDGE ( 'NONE', *, *, #2016, .F. ) ;
#7104=DIRECTION ( 'NONE',  ( -0.8746197071345569451, 0.4848096202550666312, 0.000000000000000000 ) ) ;
#7110=CARTESIAN_POINT ( 'NONE',  ( 58.00000000000000711, -2.249290599286309256, 77.19766410831374515 ) ) ;
#7118=CARTESIAN_POINT ( 'NONE',  ( 70.13889364076312916, -3.720050473604477936, 76.00117364557129918 ) ) ;
#7121=AXIS2_PLACEMENT_3D ( 'NONE', #8781, #13557, #4013 ) ;
#7129=DIRECTION ( 'NONE',  ( 0.8746197071345569451, -0.4848096202550666312, 0.000000000000000000 ) ) ;
#7130=ORIENTED_EDGE ( 'NONE', *, *, #1043, .F. ) ;
#7135=CARTESIAN_POINT ( 'NONE',  ( 65.32328153643977942, -11.87131781769073058, 75.71655242319833690 ) ) ;
#7139=AXIS2_PLACEMENT_3D ( 'NONE', #7522, #8820, #4124 ) ;
#7150=DIRECTION ( 'NONE',  ( -0.000000000000000000, 0.000000000000000000, -1.000000000000000000 ) ) ;
#7153=EDGE_CURVE ( 'NONE', #3379, #14082, #11998, .T. ) ;
#7155=CARTESIAN_POINT ( 'NONE',  ( 70.08251421541277182, -3.500407835281747371, 72.53991591819000462 ) ) ;
#7162=ORIENTED_EDGE ( 'NONE', *, *, #10485, .T. ) ;
#7164=EDGE_CURVE ( 'NONE', #1600, #7233, #5399, .T. ) ;
#7168=CYLINDRICAL_SURFACE ( 'NONE', #7665, 0.7892041907098262810 ) ;
#7170=CIRCLE ( 'NONE', #14536, 0.9999999999999957812 ) ;
#7180=DIRECTION ( 'NONE',  ( 0.000000000000000000, 0.000000000000000000, 1.000000000000000000 ) ) ;
#7188=AXIS2_PLACEMENT_3D ( 'NONE', #7967, #6725, #6646 ) ;
#7190=CARTESIAN_POINT ( 'NONE',  ( 60.40269930420516431, 2.204737408716291647, 60.61639468829817190 ) ) ;
#7200=VERTEX_POINT ( 'NONE', #12038 ) ;
#7204=VERTEX_POINT ( 'NONE', #14781 ) ;
#7206=VERTEX_POINT ( 'NONE', #1849 ) ;
#7208=CARTESIAN_POINT ( 'NONE',  ( 76.30169691776963248, -7.820670586471449859, 76.19766410831374515 ) ) ;
#7209=DIRECTION ( 'NONE',  ( -0.8746197071345571672, 0.4848096202550659650, 0.000000000000000000 ) ) ;
#7210=ADVANCED_FACE ( 'NONE', ( #11168 ), #9425, .F. ) ;
#7211=ADVANCED_FACE ( 'NONE', ( #13938 ), #10630, .F. ) ;
#7214=ORIENTED_EDGE ( 'NONE', *, *, #14373, .F. ) ;
#7218=ORIENTED_EDGE ( 'NONE', *, *, #9044, .F. ) ;
#7220=CARTESIAN_POINT ( 'NONE',  ( 64.94578693130894465, -11.37100417537640951, 76.92716210679893152 ) ) ;
#7227=EDGE_LOOP ( 'NONE', ( #11761, #1984 ) ) ;
#7229=LINE ( 'NONE', #9553, #6690 ) ;
#7233=VERTEX_POINT ( 'NONE', #9403 ) ;
#7236=DIRECTION ( 'NONE',  ( 0.000000000000000000, 0.000000000000000000, 1.000000000000000000 ) ) ;
#7249=VERTEX_POINT ( 'NONE', #14017 ) ;
#7254=CARTESIAN_POINT ( 'NONE',  ( 52.42117158417902800, -3.175556148104785592, 62.84860122826521689 ) ) ;
#7260=FACE_OUTER_BOUND ( 'NONE', #1528, .T. ) ;
#7265=CARTESIAN_POINT ( 'NONE',  ( 62.80358567007132820, -3.842053655357405173, 48.51982618741349285 ) ) ;
#7266=CARTESIAN_POINT ( 'NONE',  ( 70.22816873311688823, -4.160343359009085695, 76.17259974762927754 ) ) ;
#7267=CARTESIAN_POINT ( 'NONE',  ( 65.51779039507005109, -10.90589748781266799, 71.21143314006940273 ) ) ;
#7274=VERTEX_POINT ( 'NONE', #2320 ) ;
#7275=DIRECTION ( 'NONE',  ( -0.000000000000000000, 0.000000000000000000, -1.000000000000000000 ) ) ;
#7281=CARTESIAN_POINT ( 'NONE',  ( 64.91667272866463634, -11.40845216726351730, 75.99502765390730019 ) ) ;
#7287=EDGE_CURVE ( 'NONE', #11327, #13307, #9715, .T. ) ;
#7290=VECTOR ( 'NONE', #10371, 1000.000000000000000 ) ;
#7293=VECTOR ( 'NONE', #948, 1000.000000000000000 ) ;
#7295=VERTEX_POINT ( 'NONE', #10708 ) ;
#7301=VECTOR ( 'NONE', #2495, 1000.000000000000000 ) ;
#7306=VECTOR ( 'NONE', #3722, 1000.000000000000000 ) ;
#7316=AXIS2_PLACEMENT_3D ( 'NONE', #3848, #7547, #13465 ) ;
#7317=ORIENTED_EDGE ( 'NONE', *, *, #7691, .T. ) ;
#7319=CARTESIAN_POINT ( 'NONE',  ( 69.44126955160255932, -2.986686531272439993, 71.69793282463490414 ) ) ;
#7323=FACE_OUTER_BOUND ( 'NONE', #2621, .T. ) ;
#7327=AXIS2_PLACEMENT_3D ( 'NONE', #4813, #12727, #9107 ) ;
#7336=CARTESIAN_POINT ( 'NONE',  ( 53.34060950309435611, 1.272953934520814734, 48.51982618741349285 ) ) ;
#7341=ORIENTED_EDGE ( 'NONE', *, *, #5328, .F. ) ;
#7342=CARTESIAN_POINT ( 'NONE',  ( 69.46221311437308543, -2.886128739015260791, 75.19766410831374515 ) ) ;
#7345=EDGE_CURVE ( 'NONE', #5924, #13763, #9514, .T. ) ;
#7346=CARTESIAN_POINT ( 'NONE',  ( 65.71319926014257362, -10.73129157630437902, 72.19766410831374515 ) ) ;
#7349=FACE_BOUND ( 'NONE', #7227, .T. ) ;
#7350=CARTESIAN_POINT ( 'NONE',  ( 69.46454297103568365, -2.294433329326446280, 73.05950274574442460 ) ) ;
#7351=ORIENTED_EDGE ( 'NONE', *, *, #3105, .T. ) ;
#7357=EDGE_CURVE ( 'NONE', #556, #1600, #4370, .T. ) ;
#7358=ORIENTED_EDGE ( 'NONE', *, *, #9516, .T. ) ;
#7362=AXIS2_PLACEMENT_3D ( 'NONE', #6112, #14111, #13112 ) ;
#7368=DIRECTION ( 'NONE',  ( 0.000000000000000000, 0.000000000000000000, 1.000000000000000000 ) ) ;
#7372=ORIENTED_EDGE ( 'NONE', *, *, #1068, .F. ) ;
#7373=CARTESIAN_POINT ( 'NONE',  ( 65.22482032124671036, -11.15177368841987793, 77.09111985363571762 ) ) ;
#7374=EDGE_LOOP ( 'NONE', ( #3795, #3883, #5891, #8525 ) ) ;
#7375=ORIENTED_EDGE ( 'NONE', *, *, #2459, .F. ) ;
#7376=DIRECTION ( 'NONE',  ( -0.8208219420614786266, 0.4549890321264269955, 0.3453061251629919726 ) ) ;
#7377=ORIENTED_EDGE ( 'NONE', *, *, #3436, .F. ) ;
#7380=ORIENTED_EDGE ( 'NONE', *, *, #9117, .F. ) ;
#7381=CARTESIAN_POINT ( 'NONE',  ( 52.83848824477699679, -4.298675648159541396, 48.51982618741349285 ) ) ;
#7387=CARTESIAN_POINT ( 'NONE',  ( 58.00000000000000711, -2.249290599286309256, 60.61639468829817190 ) ) ;
#7394=CARTESIAN_POINT ( 'NONE',  ( 65.70833467347884493, -11.75568048844567848, 72.37168010940773399 ) ) ;
#7411=AXIS2_PLACEMENT_3D ( 'NONE', #2723, #1126, #9375 ) ;
#7412=CIRCLE ( 'NONE', #4953, 0.9999999999999977796 ) ;
#7419=DIRECTION ( 'NONE',  ( -0.8746197071345569451, 0.4848096202550666312, 0.000000000000000000 ) ) ;
#7420=CARTESIAN_POINT ( 'NONE',  ( 69.45904386152527366, -2.940328655257759216, 75.56077421381992565 ) ) ;
#7422=CARTESIAN_POINT ( 'NONE',  ( 65.03642989375747163, -11.30142140009759544, 71.40617678772515831 ) ) ;
#7430=CIRCLE ( 'NONE', #13562, 1.000000000000002665 ) ;
#7440=CARTESIAN_POINT ( 'NONE',  ( 58.00000000000000711, -2.249290599286309256, 82.40005259842790508 ) ) ;
#7447=EDGE_CURVE ( 'NONE', #13057, #3099, #10034, .T. ) ;
#7459=CARTESIAN_POINT ( 'NONE',  ( 58.00000000000000711, -2.249290599286309256, 76.19766410831374515 ) ) ;
#7474=EDGE_LOOP ( 'NONE', ( #2143, #12511, #14303, #7857 ) ) ;
#7475=AXIS2_PLACEMENT_3D ( 'NONE', #7603, #5143, #377 ) ;
#7477=DIRECTION ( 'NONE',  ( -0.8746197071345569451, 0.4848096202550666312, 0.000000000000000000 ) ) ;
#7479=CARTESIAN_POINT ( 'NONE',  ( 58.00000000000000711, -2.249290599286309256, 87.40005259842790508 ) ) ;
#7480=LINE ( 'NONE', #1768, #12106 ) ;
#7481=CARTESIAN_POINT ( 'NONE',  ( 66.92402464212069901, -2.249290599286309256, 39.50000000000012790 ) ) ;
#7483=CARTESIAN_POINT ( 'NONE',  ( 56.28732689558331259, 3.089731932287651084, 48.51982618741349285 ) ) ;
#7493=CARTESIAN_POINT ( 'NONE',  ( 58.00000000000000711, -2.249290599286309256, 39.50000000000012790 ) ) ;
#7497=DIRECTION ( 'NONE',  ( -0.8746197071345572782, 0.4848096202550659650, 0.000000000000000000 ) ) ;
#7502=ORIENTED_EDGE ( 'NONE', *, *, #5283, .F. ) ;
#7522=CARTESIAN_POINT ( 'NONE',  ( 118.5627027169299765, -35.81974489651393156, 54.40673322733725570 ) ) ;
#7523=VECTOR ( 'NONE', #2011, 1000.000000000000000 ) ;
#7537=DIRECTION ( 'NONE',  ( 0.000000000000000000, 0.000000000000000000, 1.000000000000000000 ) ) ;
#7547=DIRECTION ( 'NONE',  ( 0.000000000000000000, 0.000000000000000000, 1.000000000000000000 ) ) ;
#7548=DIRECTION ( 'NONE',  ( 0.000000000000000000, 0.000000000000000000, 1.000000000000000000 ) ) ;
#7549=DIRECTION ( 'NONE',  ( 0.8746197071345571672, -0.4848096202550661316, 0.000000000000000000 ) ) ;
#7552=DIRECTION ( 'NONE',  ( 0.000000000000000000, 0.000000000000000000, 1.000000000000000000 ) ) ;
#7553=CIRCLE ( 'NONE', #909, 4.000000000000003553 ) ;
#7560=CARTESIAN_POINT ( 'NONE',  ( 54.00000000000000711, -2.249290599286310588, -38.00000000000012079 ) ) ;
#7561=CARTESIAN_POINT ( 'NONE',  ( 50.19487218104683990, 2.077162398607073079, 39.50000000000012790 ) ) ;
#7562=ORIENTED_EDGE ( 'NONE', *, *, #12949, .F. ) ;
#7564=CIRCLE ( 'NONE', #9262, 1.000000000000000888 ) ;
#7565=DIRECTION ( 'NONE',  ( -0.000000000000000000, 0.000000000000000000, -1.000000000000000000 ) ) ;
#7566=DIRECTION ( 'NONE',  ( 0.000000000000000000, 0.000000000000000000, 1.000000000000000000 ) ) ;
#7571=AXIS2_PLACEMENT_3D ( 'NONE', #3577, #2581, #9279 ) ;
#7586=ORIENTED_EDGE ( 'NONE', *, *, #4527, .F. ) ;
#7591=ORIENTED_EDGE ( 'NONE', *, *, #8292, .F. ) ;
#7595=AXIS2_PLACEMENT_3D ( 'NONE', #14556, #7552, #12320 ) ;
#7596=DIRECTION ( 'NONE',  ( 0.8208219420614786266, -0.4549890321264269955, -0.3453061251629919726 ) ) ;
#7600=ORIENTED_EDGE ( 'NONE', *, *, #2199, .F. ) ;
#7603=CARTESIAN_POINT ( 'NONE',  ( 54.03086304124234829, 0.8903401505190762233, 60.61639468829817190 ) ) ;
#7606=VERTEX_POINT ( 'NONE', #11521 ) ;
#7609=CARTESIAN_POINT ( 'NONE',  ( 57.51704887355756313, 3.283153786997079049, 54.56811043785582882 ) ) ;
#7612=DIRECTION ( 'NONE',  ( 0.000000000000000000, 0.000000000000000000, 1.000000000000000000 ) ) ;
#7626=CARTESIAN_POINT ( 'NONE',  ( 65.08771336141364827, -11.27259367992862416, 72.26839924292039541 ) ) ;
#7628=ADVANCED_FACE ( 'NONE', ( #4445 ), #10779, .T. ) ;
#7654=VERTEX_POINT ( 'NONE', #9069 ) ;
#7661=CIRCLE ( 'NONE', #10363, 0.7892041907098262810 ) ;
#7665=AXIS2_PLACEMENT_3D ( 'NONE', #13168, #6025, #7477 ) ;
#7672=EDGE_CURVE ( 'NONE', #1762, #13307, #11603, .T. ) ;
#7678=AXIS2_PLACEMENT_3D ( 'NONE', #14288, #10526, #11748 ) ;
#7680=DIRECTION ( 'NONE',  ( 0.8746197071345572782, -0.4848096202550659650, -0.000000000000000000 ) ) ;
#7688=CARTESIAN_POINT ( 'NONE',  ( 52.25109540565180311, -2.012892184189034595, 48.51982618741349285 ) ) ;
#7691=EDGE_CURVE ( 'NONE', #13591, #13103, #6328, .T. ) ;
#7692=CARTESIAN_POINT ( 'NONE',  ( 53.04398595309534414, -1.224959495890951100, 48.51982618741349285 ) ) ;
#7697=AXIS2_PLACEMENT_3D ( 'NONE', #1903, #14681, #9931 ) ;
#7702=ORIENTED_EDGE ( 'NONE', *, *, #2367, .T. ) ;
#7706=CARTESIAN_POINT ( 'NONE',  ( 66.38598137497019991, -11.47113225237461087, 72.19766410831374515 ) ) ;
#7707=CARTESIAN_POINT ( 'NONE',  ( 69.32504094576864873, -4.037435678230563596, 77.18389507655805915 ) ) ;
#7711=ORIENTED_EDGE ( 'NONE', *, *, #30, .F. ) ;
#7715=ORIENTED_EDGE ( 'NONE', *, *, #8363, .F. ) ;
#7719=DIRECTION ( 'NONE',  ( -0.8746197071345576113, 0.4848096202550652989, 0.000000000000000000 ) ) ;
#7724=DIRECTION ( 'NONE',  ( 0.4848096202550659650, 0.8746197071345572782, 0.000000000000000000 ) ) ;
#7725=FACE_BOUND ( 'NONE', #8032, .T. ) ;
#7726=EDGE_CURVE ( 'NONE', #1886, #9351, #3455, .T. ) ;
#7728=ORIENTED_EDGE ( 'NONE', *, *, #30, .T. ) ;
#7730=EDGE_LOOP ( 'NONE', ( #6992, #8224, #3550, #7502 ) ) ;
#7731=DIRECTION ( 'NONE',  ( 0.000000000000000000, 0.000000000000000000, 1.000000000000000000 ) ) ;
#7732=DIRECTION ( 'NONE',  ( 0.000000000000000000, 0.000000000000000000, 1.000000000000000000 ) ) ;
#7746=ORIENTED_EDGE ( 'NONE', *, *, #1941, .F. ) ;
#7749=ORIENTED_EDGE ( 'NONE', *, *, #11660, .F. ) ;
#7751=CARTESIAN_POINT ( 'NONE',  ( 60.34603303165619792, -7.282908750500069139, 60.61639468829817190 ) ) ;
#7755=ORIENTED_EDGE ( 'NONE', *, *, #4092, .F. ) ;
#7765=TOROIDAL_SURFACE ( 'NONE', #1374, 12.46463184759105047, 1.000000000000000000 ) ;
#7768=CARTESIAN_POINT ( 'NONE',  ( 71.15942379059755751, -15.26044865788734484, 73.19766410831374515 ) ) ;
#7770=ORIENTED_EDGE ( 'NONE', *, *, #6065, .F. ) ;
#7777=EDGE_LOOP ( 'NONE', ( #865, #4800, #3052, #9549 ) ) ;
#7779=CARTESIAN_POINT ( 'NONE',  ( 65.51035252688646437, -10.91538014501780651, 72.13738083359044140 ) ) ;
#7782=CARTESIAN_POINT ( 'NONE',  ( 63.03271294676726910, -4.597264848142483373, 48.51982618741349285 ) ) ;
#7783=ORIENTED_EDGE ( 'NONE', *, *, #8348, .F. ) ;
#7784=CARTESIAN_POINT ( 'NONE',  ( 69.46451092899815194, -2.309308060028171017, 72.92418198763061810 ) ) ;
#7788=ORIENTED_EDGE ( 'NONE', *, *, #14583, .T. ) ;
#7793=VERTEX_POINT ( 'NONE', #11982 ) ;
#7799=CARTESIAN_POINT ( 'NONE',  ( 63.00747169918385993, -1.516790343742004055, 48.51982618741349285 ) ) ;
#7805=ORIENTED_EDGE ( 'NONE', *, *, #9296, .T. ) ;
#7806=DIRECTION ( 'NONE',  ( 0.000000000000000000, 0.000000000000000000, 1.000000000000000000 ) ) ;
#7812=ORIENTED_EDGE ( 'NONE', *, *, #10897, .T. ) ;
#7816=DIRECTION ( 'NONE',  ( 0.000000000000000000, 0.000000000000000000, 1.000000000000000000 ) ) ;
#7833=CYLINDRICAL_SURFACE ( 'NONE', #2159, 0.7892041907098261699 ) ;
#7837=CARTESIAN_POINT ( 'NONE',  ( 65.70654796114106944, -11.75627201178154912, 76.02260248133795528 ) ) ;
#7845=ORIENTED_EDGE ( 'NONE', *, *, #6605, .T. ) ;
#7846=CARTESIAN_POINT ( 'NONE',  ( 49.07597535787931520, -2.249290599286309256, 47.51982618741348574 ) ) ;
#7853=AXIS2_PLACEMENT_3D ( 'NONE', #13328, #12102, #6189 ) ;
#7854=AXIS2_PLACEMENT_3D ( 'NONE', #3096, #4170, #8868 ) ;
#7857=ORIENTED_EDGE ( 'NONE', *, *, #8846, .F. ) ;
#7872=LINE ( 'NONE', #12564, #7523 ) ;
#7883=LINE ( 'NONE', #12577, #1751 ) ;
#7893=LINE ( 'NONE', #12588, #8862 ) ;
#7905=DIRECTION ( 'NONE',  ( -0.8746197071345572782, 0.4848096202550660205, 0.000000000000000000 ) ) ;
#7907=FACE_OUTER_BOUND ( 'NONE', #9721, .T. ) ;
#7911=CYLINDRICAL_SURFACE ( 'NONE', #293, 5.496540510819668768 ) ;
#7914=ORIENTED_EDGE ( 'NONE', *, *, #2779, .T. ) ;
#7920=CARTESIAN_POINT ( 'NONE',  ( 70.46453521882889959, -2.298370886119723622, 75.19766410831374515 ) ) ;
#7922=ORIENTED_EDGE ( 'NONE', *, *, #10733, .T. ) ;
#7927=VECTOR ( 'NONE', #1470, 999.9999999999998863 ) ;
#7936=CARTESIAN_POINT ( 'NONE',  ( 69.46189398880601118, -2.505105728916043883, 76.08256302136429383 ) ) ;
#7958=CARTESIAN_POINT ( 'NONE',  ( 55.17185982823698964, 2.720345114498381456, 48.51982618741349285 ) ) ;
#7967=CARTESIAN_POINT ( 'NONE',  ( 53.04398595309534414, -1.224959495890951100, 60.61639468829817190 ) ) ;
#7975=CARTESIAN_POINT ( 'NONE',  ( 69.97972559857382180, -3.172990593254279457, 75.19766410831374515 ) ) ;
#7981=ORIENTED_EDGE ( 'NONE', *, *, #8104, .T. ) ;
#7982=DIRECTION ( 'NONE',  ( 0.7398406760702320728, 0.6727821148276328378, 0.000000000000000000 ) ) ;
#7984=FACE_OUTER_BOUND ( 'NONE', #1370, .T. ) ;
#7986=DIRECTION ( 'NONE',  ( -0.8746197071345570562, 0.4848096202550662981, 0.000000000000000000 ) ) ;
#7988=CARTESIAN_POINT ( 'NONE',  ( 9.211295467215947497, 29.36814620404575038, 75.19766410831374515 ) ) ;
#7995=CARTESIAN_POINT ( 'NONE',  ( 53.41380296247595538, -0.1096349785133995947, 48.51982618741349285 ) ) ;
#7999=EDGE_CURVE ( 'NONE', #7249, #1762, #12986, .T. ) ;
#8015=ORIENTED_EDGE ( 'NONE', *, *, #10928, .T. ) ;
#8029=FACE_OUTER_BOUND ( 'NONE', #454, .T. ) ;
#8032=EDGE_LOOP ( 'NONE', ( #11272, #5985, #11759, #12759, #14977, #5197, #4141, #14686, #6606, #6163, #10594, #3299, #5083, #2759, #10945, #13398, #10315, #6813, #6131, #10768, #3437, #6756, #2103, #7702, #7358, #1064, #3074, #5137, #14367, #13846, #8953, #7805, #11816, #14641, #2454 ) ) ;
#8040=LINE ( 'NONE', #5817, #7293 ) ;
#8043=DIRECTION ( 'NONE',  ( 0.000000000000000000, 0.000000000000000000, 1.000000000000000000 ) ) ;
#8044=EDGE_CURVE ( 'NONE', #2182, #14878, #3585, .T. ) ;
#8048=FACE_OUTER_BOUND ( 'NONE', #13300, .T. ) ;
#8053=CIRCLE ( 'NONE', #6342, 0.7892041907098259479 ) ;
#8063=AXIS2_PLACEMENT_3D ( 'NONE', #13581, #12357, #3963 ) ;
#8065=EDGE_LOOP ( 'NONE', ( #4670, #6724, #7770, #6457, #4775, #6302, #14595, #7098, #1306, #959, #5558, #10172, #14319, #4303, #6677, #1590, #8393, #13710, #2777, #8501, #8228, #277, #7749, #4381, #7218, #5969, #12060, #12043, #900, #5006, #8859, #2828, #5085, #4354, #6978 ) ) ;
#8069=CARTESIAN_POINT ( 'NONE',  ( 120.7275739462170918, -41.59316888568430670, 52.68020260152231060 ) ) ;
#8074=CARTESIAN_POINT ( 'NONE',  ( 76.14589960879430919, -7.734310727912411920, 75.19766410831374515 ) ) ;
#8079=DIRECTION ( 'NONE',  ( 0.8746197071345576113, -0.4848096202550652434, 0.000000000000000000 ) ) ;
#8081=EDGE_LOOP ( 'NONE', ( #10568, #12350, #12933, #10842, #13039 ) ) ;
#8085=DIRECTION ( 'NONE',  ( 1.000000000000000000, 0.000000000000000000, 0.000000000000000000 ) ) ;
#8090=CARTESIAN_POINT ( 'NONE',  ( 69.37724578219226146, -3.713350840992164947, 72.17980951935048495 ) ) ;
#8091=EDGE_CURVE ( 'NONE', #12939, #9315, #416, .T. ) ;
#8093=DIRECTION ( 'NONE',  ( -0.000000000000000000, 0.000000000000000000, -1.000000000000000000 ) ) ;
#8101=EDGE_LOOP ( 'NONE', ( #7981, #14151 ) ) ;
#8104=EDGE_CURVE ( 'NONE', #11686, #9304, #4340, .T. ) ;
#8111=ADVANCED_FACE ( 'NONE', ( #10672 ), #6212, .T. ) ;
#8124=CARTESIAN_POINT ( 'NONE',  ( 76.63070922904938698, -6.859691020777852977, 75.19766410831374515 ) ) ;
#8145=EDGE_CURVE ( 'NONE', #13687, #5691, #10575, .T. ) ;
#8148=ORIENTED_EDGE ( 'NONE', *, *, #14675, .F. ) ;
#8155=ORIENTED_EDGE ( 'NONE', *, *, #4132, .F. ) ;
#8164=CARTESIAN_POINT ( 'NONE',  ( 70.14622571237704562, -3.746881330724391557, 72.37272573528950659 ) ) ;
#8165=ORIENTED_EDGE ( 'NONE', *, *, #9454, .T. ) ;
#8170=DIRECTION ( 'NONE',  ( -0.8208219420614808470, 0.4549890321264226656, 0.3453061251629923611 ) ) ;
#8178=FACE_OUTER_BOUND ( 'NONE', #1290, .T. ) ;
#8180=ORIENTED_EDGE ( 'NONE', *, *, #4763, .F. ) ;
#8182=DIRECTION ( 'NONE',  ( 0.8746197071345572782, -0.4848096202550659650, 0.000000000000000000 ) ) ;
#8183=DIRECTION ( 'NONE',  ( -0.000000000000000000, 0.000000000000000000, -1.000000000000000000 ) ) ;
#8186=AXIS2_PLACEMENT_3D ( 'NONE', #10710, #5017, #9722 ) ;
#8189=DIRECTION ( 'NONE',  ( 0.000000000000000000, 0.000000000000000000, 1.000000000000000000 ) ) ;
#8193=DIRECTION ( 'NONE',  ( -0.3020115420618248447, 0.1674077314120184512, -0.9384901064608619503 ) ) ;
#8203=VECTOR ( 'NONE', #11434, 1000.000000000000000 ) ;
#8210=CARTESIAN_POINT ( 'NONE',  ( 50.07597535787931520, -2.249290599286309256, 48.51982618741349285 ) ) ;
#8211=CARTESIAN_POINT ( 'NONE',  ( 54.03086304124234829, 0.8903401505190762233, 60.61639468829817190 ) ) ;
#8212=CARTESIAN_POINT ( 'NONE',  ( 61.57572300660984865, -8.804762498903286883, 76.19766410831374515 ) ) ;
#8217=ORIENTED_EDGE ( 'NONE', *, *, #1040, .F. ) ;
#8220=EDGE_CURVE ( 'NONE', #4043, #211, #12575, .T. ) ;
#8221=DIRECTION ( 'NONE',  ( -0.7152862910730209967, -0.6988315403607663345, 0.000000000000000000 ) ) ;
#8224=ORIENTED_EDGE ( 'NONE', *, *, #12062, .T. ) ;
#8225=CARTESIAN_POINT ( 'NONE',  ( 65.27061521436114333, -11.12190849844603058, 76.21551869727603901 ) ) ;
#8226=DIRECTION ( 'NONE',  ( 0.8746197071345573892, -0.4848096202550657985, 0.000000000000000000 ) ) ;
#8228=ORIENTED_EDGE ( 'NONE', *, *, #1010, .F. ) ;
#8229=EDGE_LOOP ( 'NONE', ( #10518, #4572, #13923, #9566 ) ) ;
#8231=CARTESIAN_POINT ( 'NONE',  ( 53.11142512232702018, -3.558169932106523881, 60.61639468829817190 ) ) ;
#8245=FACE_OUTER_BOUND ( 'NONE', #14090, .T. ) ;
#8255=CARTESIAN_POINT ( 'NONE',  ( 53.54504563787001814, -4.650271872399136086, 62.84860122826521689 ) ) ;
#8276=DIRECTION ( 'NONE',  ( 0.000000000000000000, 0.000000000000000000, 1.000000000000000000 ) ) ;
#8282=AXIS2_PLACEMENT_3D ( 'NONE', #5796, #14175, #2242 ) ;
#8292=EDGE_CURVE ( 'NONE', #117, #13103, #10070, .T. ) ;
#8296=AXIS2_PLACEMENT_3D ( 'NONE', #14511, #8658, #12501 ) ;
#8298=CARTESIAN_POINT ( 'NONE',  ( 65.13162939602318602, -11.91918766459985335, 75.19766410831374515 ) ) ;
#8299=CYLINDRICAL_SURFACE ( 'NONE', #7052, 11.46463184759105403 ) ;
#8301=AXIS2_PLACEMENT_3D ( 'NONE', #9748, #1427, #1504 ) ;
#8305=ADVANCED_FACE ( 'NONE', ( #7260 ), #1227, .T. ) ;
#8315=EDGE_LOOP ( 'NONE', ( #13433, #4758, #9639, #15039 ) ) ;
#8322=CARTESIAN_POINT ( 'NONE',  ( 55.08546260466144417, 2.477934215446290445, 54.56811043785582882 ) ) ;
#8332=DIRECTION ( 'NONE',  ( 0.000000000000000000, 0.000000000000000000, 1.000000000000000000 ) ) ;
#8333=EDGE_CURVE ( 'NONE', #59, #2925, #13275, .T. ) ;
#8334=EDGE_LOOP ( 'NONE', ( #15150, #772, #12618, #14193 ) ) ;
#8336=ORIENTED_EDGE ( 'NONE', *, *, #8388, .F. ) ;
#8345=DIRECTION ( 'NONE',  ( -0.8746197071345569451, 0.4848096202550666312, 0.000000000000000000 ) ) ;
#8348=EDGE_CURVE ( 'NONE', #10484, #11185, #5401, .T. ) ;
#8352=EDGE_LOOP ( 'NONE', ( #12333, #4470, #2075, #2876, #8387 ) ) ;
#8354=FACE_OUTER_BOUND ( 'NONE', #13717, .T. ) ;
#8356=DIRECTION ( 'NONE',  ( -0.8208219420614786266, 0.4549890321264268844, 0.3453061251629920281 ) ) ;
#8357=CARTESIAN_POINT ( 'NONE',  ( 70.25043121783370736, -4.317737931693936382, 76.19766410831374515 ) ) ;
#8358=CARTESIAN_POINT ( 'NONE',  ( 65.22587406926737685, -11.15092874177724980, 71.30368058120426156 ) ) ;
#8361=CYLINDRICAL_SURFACE ( 'NONE', #7571, 1.000000000000005329 ) ;
#8363=EDGE_CURVE ( 'NONE', #5234, #3379, #3650, .T. ) ;
#8366=CARTESIAN_POINT ( 'NONE',  ( 58.14816640453862107, 2.809303687574978614, 60.61639468829817190 ) ) ;
#8371=CARTESIAN_POINT ( 'NONE',  ( 65.62087295291071598, -10.81524950655579786, 76.23790561730409365 ) ) ;
#8379=ORIENTED_EDGE ( 'NONE', *, *, #4601, .F. ) ;
#8381=EDGE_CURVE ( 'NONE', #10163, #2925, #4416, .T. ) ;
#8383=FACE_OUTER_BOUND ( 'NONE', #2552, .T. ) ;
#8387=ORIENTED_EDGE ( 'NONE', *, *, #2868, .F. ) ;
#8388=EDGE_CURVE ( 'NONE', #11544, #2180, #12023, .T. ) ;
#8393=ORIENTED_EDGE ( 'NONE', *, *, #9520, .F. ) ;
#8398=AXIS2_PLACEMENT_3D ( 'NONE', #4388, #13775, #12629 ) ;
#8411=EDGE_CURVE ( 'NONE', #1886, #12128, #10324, .T. ) ;
#8423=CIRCLE ( 'NONE', #10375, 0.7892041907098262810 ) ;
#8427=LINE ( 'NONE', #9430, #3004 ) ;
#8433=VECTOR ( 'NONE', #7596, 999.9999999999998863 ) ;
#8435=CARTESIAN_POINT ( 'NONE',  ( 69.37744794823258587, -3.711917656928557463, 76.21513011789701864 ) ) ;
#8451=B_SPLINE_CURVE_WITH_KNOTS ( 'NONE', 3,
 ( #8629, #11304, #12630, #5629, #11534, #7936, #6695, #3082, #2077, #13706, #10238, #993, #6767, #14931, #10089, #7707, #11233, #3313 ),
 .UNSPECIFIED., .F., .F.,
 ( 4, 2, 2, 2, 2, 2, 2, 2, 4 ),
 ( 0.000000000000000000, 0.0003958370570530562473, 0.0007916741141061124946, 0.001187511171159168688, 0.001583348228212224989, 0.001979185285265281074, 0.002375022342318337375, 0.002770859399371394111, 0.003166696456424448677 ),
 .UNSPECIFIED. ) ;
#8452=ORIENTED_EDGE ( 'NONE', *, *, #14320, .F. ) ;
#8459=EDGE_LOOP ( 'NONE', ( #13428, #10113, #3316, #3679 ) ) ;
#8462=LINE ( 'NONE', #8523, #8768 ) ;
#8481=ORIENTED_EDGE ( 'NONE', *, *, #14855, .T. ) ;
#8495=CYLINDRICAL_SURFACE ( 'NONE', #7853, 0.7892041907098262810 ) ;
#8499=EDGE_CURVE ( 'NONE', #12128, #2824, #6883, .T. ) ;
#8501=ORIENTED_EDGE ( 'NONE', *, *, #3944, .F. ) ;
#8502=DIRECTION ( 'NONE',  ( 0.8208219420614780715, -0.4549890321264283277, -0.3453061251629916950 ) ) ;
#8504=CARTESIAN_POINT ( 'NONE',  ( 69.41360828637785119, -3.335076845702578119, 76.94374568549258697 ) ) ;
#8506=CARTESIAN_POINT ( 'NONE',  ( 65.67990869784712515, -11.76427225047157776, 72.39415457105613427 ) ) ;
#8523=CARTESIAN_POINT ( 'NONE',  ( 76.78650653802468184, -6.946050879336882922, 75.19766410831374515 ) ) ;
#8524=CIRCLE ( 'NONE', #639, 0.7892041907098262810 ) ;
#8525=ORIENTED_EDGE ( 'NONE', *, *, #3409, .T. ) ;
#8533=VERTEX_POINT ( 'NONE', #1782 ) ;
#8540=AXIS2_PLACEMENT_3D ( 'NONE', #9929, #14604, #4053 ) ;
#8553=ORIENTED_EDGE ( 'NONE', *, *, #10191, .F. ) ;
#8554=CARTESIAN_POINT ( 'NONE',  ( 62.30678795759143185, -4.906903613034745426, 48.51982618741349285 ) ) ;
#8558=VECTOR ( 'NONE', #11791, 1000.000000000000000 ) ;
#8564=VERTEX_POINT ( 'NONE', #4306 ) ;
#8567=DIRECTION ( 'NONE',  ( 0.000000000000000000, 0.000000000000000000, 1.000000000000000000 ) ) ;
#8568=DIRECTION ( 'NONE',  ( 0.9111637130653279515, 0.4120445218577777902, 0.000000000000000000 ) ) ;
#8571=CARTESIAN_POINT ( 'NONE',  ( 69.45041322604760126, -2.827919977413038133, 76.54331634761751957 ) ) ;
#8579=UNCERTAINTY_MEASURE_WITH_UNIT (LENGTH_MEASURE( 1.000000000000000082E-05 ), #854, 'distance_accuracy_value', 'NONE');
#8582=FACE_OUTER_BOUND ( 'NONE', #4792, .T. ) ;
#8583=VERTEX_POINT ( 'NONE', #6544 ) ;
#8586=TOROIDAL_SURFACE ( 'NONE', #10561, 7.924024642120688355, 1.000000000000000000 ) ;
#8594=AXIS2_PLACEMENT_3D ( 'NONE', #185, #10578, #6039 ) ;
#8605=ORIENTED_EDGE ( 'NONE', *, *, #8411, .F. ) ;
#8611=DIRECTION ( 'NONE',  ( 0.8746197071345573892, -0.4848096202550657430, 0.000000000000000000 ) ) ;
#8612=CARTESIAN_POINT ( 'NONE',  ( 62.88869237673507229, 0.3854521819929429549, 48.51982618741349285 ) ) ;
#8614=ORIENTED_EDGE ( 'NONE', *, *, #5413, .T. ) ;
#8619=VERTEX_POINT ( 'NONE', #4549 ) ;
#8621=CARTESIAN_POINT ( 'NONE',  ( 72.26742264675378635, -14.73126838498887281, 76.19766410831374515 ) ) ;
#8629=CARTESIAN_POINT ( 'NONE',  ( 69.46454297106444642, -2.294433322023680333, 75.19766410831374515 ) ) ;
#8637=DIRECTION ( 'NONE',  ( 0.000000000000000000, 0.000000000000000000, -1.000000000000000000 ) ) ;
#8638=CARTESIAN_POINT ( 'NONE',  ( 63.03271294676726910, -4.597264848142476268, 54.56811043785582882 ) ) ;
#8640=CARTESIAN_POINT ( 'NONE',  ( 64.68848588106907016, -11.56114324328357057, 71.69770485003853366 ) ) ;
#8658=DIRECTION ( 'NONE',  ( 0.000000000000000000, 0.000000000000000000, -1.000000000000000000 ) ) ;
#8670=EDGE_CURVE ( 'NONE', #7200, #3379, #2713, .T. ) ;
#8672=DIRECTION ( 'NONE',  ( -0.000000000000000000, 0.000000000000000000, -1.000000000000000000 ) ) ;
#8677=ADVANCED_BREP_SHAPE_REPRESENTATION ( '', ( #14200, #6315 ), #4840 ) ;
#8678=DIRECTION ( 'NONE',  ( 0.8208219420614786266, -0.4549890321264269399, -0.3453061251629920836 ) ) ;
#8680=EDGE_LOOP ( 'NONE', ( #10441, #807, #11602, #5263 ) ) ;
#8687=EDGE_LOOP ( 'NONE', ( #15141, #13635, #11162 ) ) ;
#8731=CARTESIAN_POINT ( 'NONE',  ( 47.97280705105441001, 3.308873213108444400, 81.40005259842790508 ) ) ;
#8732=EDGE_CURVE ( 'NONE', #3976, #6117, #11803, .T. ) ;
#8733=ORIENTED_EDGE ( 'NONE', *, *, #1829, .F. ) ;
#8740=CARTESIAN_POINT ( 'NONE',  ( 58.00000000000000711, -2.249290599286309256, 82.40005259842790508 ) ) ;
#8742=ORIENTED_EDGE ( 'NONE', *, *, #14496, .T. ) ;
#8744=CARTESIAN_POINT ( 'NONE',  ( 56.25419740419757630, 3.022649838004307199, 60.61639468829817190 ) ) ;
#8747=EDGE_CURVE ( 'NONE', #2925, #211, #12045, .T. ) ;
#8752=FACE_OUTER_BOUND ( 'NONE', #2774, .T. ) ;
#8760=VERTEX_POINT ( 'NONE', #3975 ) ;
#8762=AXIS2_PLACEMENT_3D ( 'NONE', #12603, #14746, #2053 ) ;
#8766=DIRECTION ( 'NONE',  ( 0.000000000000000000, 0.000000000000000000, 1.000000000000000000 ) ) ;
#8768=VECTOR ( 'NONE', #1287, 1000.000000000000000 ) ;
#8769=CARTESIAN_POINT ( 'NONE',  ( 70.17742216864051841, -3.884085244343386645, 76.08660377794682006 ) ) ;
#8770=CARTESIAN_POINT ( 'NONE',  ( 61.93276294469178822, -4.429256696798314685, 86.40005259842790508 ) ) ;
#8779=VERTEX_POINT ( 'NONE', #657 ) ;
#8781=CARTESIAN_POINT ( 'NONE',  ( 62.70356846721307420, -0.3817325368051065482, 60.61639468829817190 ) ) ;
#8784=DIRECTION ( 'NONE',  ( 0.8746197071345503948, -0.4848096202550782885, 0.000000000000000000 ) ) ;
#8786=CLOSED_SHELL ( 'NONE', ( #6832, #9942, #14353, #10896, #7628, #9801, #8305, #13222, #12515, #7014, #3945, #140, #11474, #1783, #8111, #4762, #6768, #9973, #9857, #610, #3169, #14987, #12932, #1610, #9099, #2650, #3855, #14404, #3168, #10473, #27, #11566, #14334, #6177, #2599, #3211, #10263, #3050, #9583, #10314, #3863, #13274, #5019, #5285, #12660, #15023, #4075, #3351, #3878, #692, #5185, #13396, #4907, #3362, #10941, #4544, #12644, #1971, #11953, #13216, #5243, #13154, #11737, #6198, #2107, #14589, #3941, #3777, #2832, #11278, #11567, #1461, #10975, #10639, #8872, #2915, #10839, #6106, #4144, #7210, #14715, #6576, #6470, #12139, #7211, #6622, #2271, #5763, #7084, #3394, #10882, #11821 ) ) ;
#8796=ORIENTED_EDGE ( 'NONE', *, *, #11092, .T. ) ;
#8807=EDGE_CURVE ( 'NONE', #11185, #10484, #14737, .T. ) ;
#8812=ORIENTED_EDGE ( 'NONE', *, *, #3318, .T. ) ;
#8818=AXIS2_PLACEMENT_3D ( 'NONE', #10651, #12809, #12647 ) ;
#8819=ORIENTED_EDGE ( 'NONE', *, *, #12258, .F. ) ;
#8820=DIRECTION ( 'NONE',  ( 0.3020115420618247892, -0.1674077314120183957, 0.9384901064608620613 ) ) ;
#8821=CARTESIAN_POINT ( 'NONE',  ( 69.46373988936370836, -2.401367963164388719, 72.55353403238311216 ) ) ;
#8822=DIRECTION ( 'NONE',  ( -0.8746197071345570562, 0.4848096202550665756, 0.000000000000000000 ) ) ;
#8823=CARTESIAN_POINT ( 'NONE',  ( 53.27389963060701916, 0.6670697996139958175, 48.51982618741349285 ) ) ;
#8841=LINE ( 'NONE', #1765, #318 ) ;
#8846=EDGE_CURVE ( 'NONE', #3165, #6912, #12435, .T. ) ;
#8848=ORIENTED_EDGE ( 'NONE', *, *, #5611, .F. ) ;
#8852=DIRECTION ( 'NONE',  ( 0.000000000000000000, 0.000000000000000000, 1.000000000000000000 ) ) ;
#8859=ORIENTED_EDGE ( 'NONE', *, *, #3828, .F. ) ;
#8862=VECTOR ( 'NONE', #12664, 1000.000000000000000 ) ;
#8864=ORIENTED_EDGE ( 'NONE', *, *, #14702, .F. ) ;
#8868=DIRECTION ( 'NONE',  ( 0.4331347858759544978, 0.9013291614411413910, 0.000000000000000000 ) ) ;
#8870=CIRCLE ( 'NONE', #44, 0.7892041907098272802 ) ;
#8872=ADVANCED_FACE ( 'NONE', ( #13371 ), #2827, .F. ) ;
#8873=EDGE_LOOP ( 'NONE', ( #3634, #10402, #9072, #858 ) ) ;
#8878=ORIENTED_EDGE ( 'NONE', *, *, #7164, .T. ) ;
#8882=EDGE_CURVE ( 'NONE', #6117, #1886, #2963, .T. ) ;
#8888=DIRECTION ( 'NONE',  ( -0.8746197071345560570, 0.4848096202550682410, 0.000000000000000000 ) ) ;
#8894=ORIENTED_EDGE ( 'NONE', *, *, #10123, .T. ) ;
#8903=CIRCLE ( 'NONE', #7188, 0.7892041907098262810 ) ;
#8904=CARTESIAN_POINT ( 'NONE',  ( 52.46774229227035136, -1.764205727211077379, 54.56811043785582882 ) ) ;
#8910=TOROIDAL_SURFACE ( 'NONE', #2282, 3.999999999999996447, 1.000000000000000000 ) ;
#8912=CARTESIAN_POINT ( 'NONE',  ( 52.46774229227035136, -1.764205727211077379, 48.51982618741349285 ) ) ;
#8927=EDGE_LOOP ( 'NONE', ( #7586, #1836, #14666, #3203 ) ) ;
#8930=CARTESIAN_POINT ( 'NONE',  ( 64.91683959679546945, -11.40731206199988890, 72.41114282892958443 ) ) ;
#8936=CARTESIAN_POINT ( 'NONE',  ( 69.46140857195989327, -2.899158388209396975, 73.01624609662880516 ) ) ;
#8943=CARTESIAN_POINT ( 'NONE',  ( 64.64681977576807981, -12.79380737173440430, 75.19766410831374515 ) ) ;
#8952=DIRECTION ( 'NONE',  ( -0.8746197071345569451, 0.4848096202550666312, 0.000000000000000000 ) ) ;
#8953=ORIENTED_EDGE ( 'NONE', *, *, #12807, .T. ) ;
#8960=ORIENTED_EDGE ( 'NONE', *, *, #230, .T. ) ;
#8975=CARTESIAN_POINT ( 'NONE',  ( 69.45693112140031644, -2.708622645674852780, 71.97298415572764441 ) ) ;
#8986=EDGE_LOOP ( 'NONE', ( #9543, #79, #5572, #9812 ) ) ;
#8991=CARTESIAN_POINT ( 'NONE',  ( 63.43853564383336874, -3.373351419973840581, 54.56811043785582882 ) ) ;
#8995=DIRECTION ( 'NONE',  ( 0.000000000000000000, 0.000000000000000000, 1.000000000000000000 ) ) ;
#8999=DIRECTION ( 'NONE',  ( -0.9971413439177307936, -0.07555885288926501853, 0.000000000000000000 ) ) ;
#9001=EDGE_CURVE ( 'NONE', #8619, #3324, #10831, .T. ) ;
#9003=DIRECTION ( 'NONE',  ( 0.4848096202550661871, 0.8746197071345573892, -0.000000000000000000 ) ) ;
#9008=CARTESIAN_POINT ( 'NONE',  ( 69.46363198353849100, -2.410414910243239728, 72.52785177043239173 ) ) ;
#9012=ORIENTED_EDGE ( 'NONE', *, *, #4950, .T. ) ;
#9014=CARTESIAN_POINT ( 'NONE',  ( 75.52271037289314393, -7.388871293676331220, 71.19766410831374515 ) ) ;
#9016=DIRECTION ( 'NONE',  ( -0.8746197071345569451, 0.4848096202550666312, 0.000000000000000000 ) ) ;
#9021=VECTOR ( 'NONE', #5584, 1000.000000000000000 ) ;
#9026=DIRECTION ( 'NONE',  ( -0.8208219420614771833, 0.4549890321264261628, 0.3453061251629969131 ) ) ;
#9044=EDGE_CURVE ( 'NONE', #7793, #13057, #9329, .T. ) ;
#9047=CARTESIAN_POINT ( 'NONE',  ( 67.15257324181105503, -7.322644791425992672, 81.40005259842790508 ) ) ;
#9054=ORIENTED_EDGE ( 'NONE', *, *, #1656, .T. ) ;
#9065=LINE ( 'NONE', #13759, #8203 ) ;
#9067=ORIENTED_EDGE ( 'NONE', *, *, #11099, .T. ) ;
#9069=CARTESIAN_POINT ( 'NONE',  ( 62.14930354033766946, 1.441842398587370067, 48.51982618741349285 ) ) ;
#9072=ORIENTED_EDGE ( 'NONE', *, *, #10558, .F. ) ;
#9079=EDGE_CURVE ( 'NONE', #5924, #117, #2194, .T. ) ;
#9080=CIRCLE ( 'NONE', #12263, 2.000000000000001776 ) ;
#9082=CARTESIAN_POINT ( 'NONE',  ( 117.5294988620952097, -39.82044691928823710, 57.22220354671985376 ) ) ;
#9084=ORIENTED_EDGE ( 'NONE', *, *, #8104, .F. ) ;
#9086=CARTESIAN_POINT ( 'NONE',  ( 65.28554636553401735, -11.88096418064013093, 72.74061878094576628 ) ) ;
#9091=CARTESIAN_POINT ( 'NONE',  ( 62.35557539207178479, -5.694598376804811402, 54.56811043785582882 ) ) ;
#9099=ADVANCED_FACE ( 'NONE', ( #3033, #7725 ), #12410, .F. ) ;
#9100=EDGE_CURVE ( 'NONE', #996, #1587, #12022, .T. ) ;
#9101=( NAMED_UNIT ( * ) PLANE_ANGLE_UNIT ( ) SI_UNIT ( $, .RADIAN. ) );
#9107=DIRECTION ( 'NONE',  ( -0.8746197071345572782, 0.4848096202550659650, 0.000000000000000000 ) ) ;
#9115=DIRECTION ( 'NONE',  ( 0.000000000000000000, 0.000000000000000000, 1.000000000000000000 ) ) ;
#9117=EDGE_CURVE ( 'NONE', #4051, #14177, #1214, .T. ) ;
#9125=B_SPLINE_CURVE_WITH_KNOTS ( 'NONE', 3,
 ( #10866, #1746, #13518, #3128, #2623, #14597, #4045, #2903, #7319, #8975, #14668, #8821, #3780, #11205, #13595, #5527 ),
 .UNSPECIFIED., .F., .F.,
 ( 4, 2, 2, 2, 2, 2, 2, 4 ),
 ( 0.000000000000000000, 0.0003911934542035802576, 0.0007823869084071605152, 0.001173580362610740719, 0.001564773816814321030, 0.002347160725221481004, 0.002738354179425079964, 0.003129547633628678924 ),
 .UNSPECIFIED. ) ;
#9142=CARTESIAN_POINT ( 'NONE',  ( 69.28051765693513175, -4.295678830383773850, 76.19766410831374515 ) ) ;
#9143=CARTESIAN_POINT ( 'NONE',  ( 4.848008884920353090, 21.49656883983473676, 73.19766410831374515 ) ) ;
#9147=ORIENTED_EDGE ( 'NONE', *, *, #10466, .T. ) ;
#9150=VECTOR ( 'NONE', #11691, 1000.000000000000000 ) ;
#9152=CYLINDRICAL_SURFACE ( 'NONE', #10068, 1.000000000000000888 ) ;
#9154=CARTESIAN_POINT ( 'NONE',  ( 63.55116547662790794, -2.088839582009629936, 48.51982618741349285 ) ) ;
#9158=VERTEX_POINT ( 'NONE', #7958 ) ;
#9162=AXIS2_PLACEMENT_3D ( 'NONE', #3420, #9115, #12498 ) ;
#9171=CYLINDRICAL_SURFACE ( 'NONE', #9188, 0.7892041907098262810 ) ;
#9175=CARTESIAN_POINT ( 'NONE',  ( 69.43268765340762627, -3.261345579701428132, 72.40030056272208014 ) ) ;
#9188=AXIS2_PLACEMENT_3D ( 'NONE', #13858, #14933, #1154 ) ;
#9189=DIRECTION ( 'NONE',  ( 0.000000000000000000, 0.000000000000000000, 1.000000000000000000 ) ) ;
#9192=CARTESIAN_POINT ( 'NONE',  ( 53.04398595309534414, -1.224959495890951100, 60.61639468829817190 ) ) ;
#9193=EDGE_CURVE ( 'NONE', #6176, #13057, #3257, .T. ) ;
#9195=EDGE_CURVE ( 'NONE', #7204, #7606, #12517, .T. ) ;
#9196=ORIENTED_EDGE ( 'NONE', *, *, #4515, .T. ) ;
#9214=ORIENTED_EDGE ( 'NONE', *, *, #11909, .F. ) ;
#9237=DIRECTION ( 'NONE',  ( 0.000000000000000000, 0.000000000000000000, 1.000000000000000000 ) ) ;
#9243=DIRECTION ( 'NONE',  ( -0.000000000000000000, -0.000000000000000000, -1.000000000000000000 ) ) ;
#9249=CARTESIAN_POINT ( 'NONE',  ( 70.25061521000239395, -4.319789889307661390, 72.19766410831373094 ) ) ;
#9255=ORIENTED_EDGE ( 'NONE', *, *, #5371, .T. ) ;
#9262=AXIS2_PLACEMENT_3D ( 'NONE', #3076, #14921, #5387 ) ;
#9266=CARTESIAN_POINT ( 'NONE',  ( 121.8927854443908103, -31.94886955507721638, 57.22220354671986087 ) ) ;
#9279=DIRECTION ( 'NONE',  ( 0.3020115420618222357, -0.1674077314120182292, 0.9384901064608630605 ) ) ;
#9286=CIRCLE ( 'NONE', #2145, 1.000000000000000888 ) ;
#9296=EDGE_CURVE ( 'NONE', #14840, #3763, #13748, .T. ) ;
#9304=VERTEX_POINT ( 'NONE', #7560 ) ;
#9307=DIRECTION ( 'NONE',  ( 0.3020115420618285085, -0.1674077314120178406, 0.9384901064608609511 ) ) ;
#9309=ORIENTED_EDGE ( 'NONE', *, *, #1881, .T. ) ;
#9310=CARTESIAN_POINT ( 'NONE',  ( 60.65595175199513278, -6.557103238384438981, 60.61639468829817190 ) ) ;
#9315=VERTEX_POINT ( 'NONE', #406 ) ;
#9316=DIRECTION ( 'NONE',  ( -0.000000000000000000, -0.000000000000000000, -1.000000000000000000 ) ) ;
#9327=CARTESIAN_POINT ( 'NONE',  ( 119.4687373431154782, -36.32196809074999777, 57.22220354671986797 ) ) ;
#9329=CIRCLE ( 'NONE', #7854, 0.7892041907098270581 ) ;
#9331=CARTESIAN_POINT ( 'NONE',  ( 58.00000000000000711, -2.249290599286311032, -49.31370849898490150 ) ) ;
#9338=FACE_OUTER_BOUND ( 'NONE', #6076, .T. ) ;
#9346=DIRECTION ( 'NONE',  ( 0.8208219420614786266, -0.4549890321264268844, -0.3453061251629920281 ) ) ;
#9351=VERTEX_POINT ( 'NONE', #5721 ) ;
#9352=DIRECTION ( 'NONE',  ( -0.8746197071345569451, 0.4848096202550666312, 0.000000000000000000 ) ) ;
#9361=ORIENTED_EDGE ( 'NONE', *, *, #14502, .T. ) ;
#9363=PRODUCT_DEFINITION_CONTEXT ( 'detailed design', #11431, 'design' ) ;
#9370=CARTESIAN_POINT ( 'NONE',  ( 65.14946943679815661, -11.22247402132563998, 76.16304653356505128 ) ) ;
#9374=EDGE_LOOP ( 'NONE', ( #2435, #150, #1635, #6138 ) ) ;
#9375=DIRECTION ( 'NONE',  ( 0.8746197071345572782, -0.4848096202550659650, 0.000000000000000000 ) ) ;
#9376=CARTESIAN_POINT ( 'NONE',  ( 64.11356537587559501, -11.94785244090458498, 82.40005259842790508 ) ) ;
#9378=CIRCLE ( 'NONE', #3714, 0.7892041907098270581 ) ;
#9379=DIRECTION ( 'NONE',  ( 0.4848096202550659650, 0.8746197071345572782, 0.000000000000000000 ) ) ;
#9396=CARTESIAN_POINT ( 'NONE',  ( 55.09646579789918519, -6.394265699299607419, 60.61639468829817190 ) ) ;
#9400=CARTESIAN_POINT ( 'NONE',  ( 76.16331730212350237, -6.600611445100788899, 72.19766410831374515 ) ) ;
#9403=CARTESIAN_POINT ( 'NONE',  ( 62.35557539207178479, -5.694598376804811402, 48.51982618741349285 ) ) ;
#9406=ORIENTED_EDGE ( 'NONE', *, *, #7287, .T. ) ;
#9412=CYLINDRICAL_SURFACE ( 'NONE', #3006, 0.7892041907098262810 ) ;
#9420=FACE_OUTER_BOUND ( 'NONE', #1138, .T. ) ;
#9425=( BOUNDED_SURFACE ( )  B_SPLINE_SURFACE ( 3, 2, ( 
 ( #547, #5253, #690 ),
 ( #7350, #4234, #11309 ),
 ( #7784, #8936, #3086 ),
 ( #1925, #846, #14854 ),
 ( #9008, #1502, #13780 ),
 ( #13712, #5553, #10898 ),
 ( #2394, #9175, #3551 ),
 ( #13861, #2238, #10477 ),
 ( #10323, #15098, #12711 ),
 ( #1235, #8090, #5946 ),
 ( #4548, #5876, #14098 ),
 ( #12946, #7094, #15017 ),
 ( #4785, #10404, #9249 ),
 ( #11459, #924, #3317 ) ),
 .UNSPECIFIED., .F., .F., .F. ) 
 B_SPLINE_SURFACE_WITH_KNOTS ( ( 4, 2, 2, 2, 2, 2, 4 ),
 ( 3, 3 ),
 ( 0.001231944704344905541, 0.001640530120327078883, 0.002049115536309252007, 0.002866286368273598256, 0.003274871784255771381, 0.003683457200237944505, 0.004500628032202290754 ),
 ( 0.000000000000000000, 1.000000000000000000 ),
 .UNSPECIFIED. ) 
 GEOMETRIC_REPRESENTATION_ITEM ( )  RATIONAL_B_SPLINE_SURFACE ( (
 ( 1.000000000000000000, 0.8606282562001420500, 1.000000000000000000),
 ( 1.000000000000000000, 0.8606242962985151124, 1.000000000000000000),
 ( 1.000000000000000000, 0.8593044206441436961, 1.000000000000000000),
 ( 1.000000000000000000, 0.8542070032140108848, 1.000000000000000000),
 ( 1.000000000000000000, 0.8503651661363297309, 1.000000000000000000),
 ( 1.000000000000000000, 0.8359148296423946078, 1.000000000000000000),
 ( 1.000000000000000000, 0.8221039232028367616, 1.000000000000000000),
 ( 1.000000000000000000, 0.7986554744406206829, 1.000000000000000000),
 ( 1.000000000000000000, 0.7902603328760277046, 1.000000000000000000),
 ( 1.000000000000000000, 0.7732499594489120609, 1.000000000000000000),
 ( 1.000000000000000000, 0.7646145331266447354, 1.000000000000000000),
 ( 1.000000000000000000, 0.7387090984038677810, 1.000000000000000000),
 ( 1.000000000000000000, 0.7216377402996817514, 1.000000000000000000),
 ( 1.000000000000000000, 0.7071067811865475727, 1.000000000000000000) ) ) 
 REPRESENTATION_ITEM ( '' )  SURFACE ( )  );
#9426=EDGE_LOOP ( 'NONE', ( #9617, #8180, #5492, #12376 ) ) ;
#9430=CARTESIAN_POINT ( 'NONE',  ( 53.27389963060701916, 0.6670697996139958175, 54.56811043785582882 ) ) ;
#9431=CIRCLE ( 'NONE', #5745, 0.7892041907098275022 ) ;
#9437=CARTESIAN_POINT ( 'NONE',  ( 69.45429961572709487, -2.741948779197806996, 76.44472825213317435 ) ) ;
#9440=CARTESIAN_POINT ( 'NONE',  ( 58.00000000000000711, -2.249290599286309256, 77.19766410831374515 ) ) ;
#9448=ORIENTED_EDGE ( 'NONE', *, *, #3944, .T. ) ;
#9450=CARTESIAN_POINT ( 'NONE',  ( 65.81665574905483140, -11.71669805552613752, 76.07128683897853705 ) ) ;
#9454=EDGE_CURVE ( 'NONE', #6287, #6894, #10250, .T. ) ;
#9477=DIRECTION ( 'NONE',  ( 0.000000000000000000, 0.000000000000000000, -1.000000000000000000 ) ) ;
#9488=EDGE_CURVE ( 'NONE', #12270, #10980, #4324, .T. ) ;
#9496=CARTESIAN_POINT ( 'NONE',  ( 117.2274873200333900, -39.65303918787621740, 56.28371344025897116 ) ) ;
#9499=AXIS2_PLACEMENT_3D ( 'NONE', #9327, #15174, #11704 ) ;
#9504=CARTESIAN_POINT ( 'NONE',  ( 58.80593636315131079, 3.245402227105440129, 60.61639468829817190 ) ) ;
#9507=CARTESIAN_POINT ( 'NONE',  ( 69.42475957733114456, -3.331272038940554570, 76.03737743669417171 ) ) ;
#9514=CIRCLE ( 'NONE', #6573, 1.000000000000000888 ) ;
#9516=EDGE_CURVE ( 'NONE', #6563, #9615, #6061, .T. ) ;
#9520=EDGE_CURVE ( 'NONE', #14454, #6912, #2374, .T. ) ;
#9528=CARTESIAN_POINT ( 'NONE',  ( 65.88651289459839688, -11.69095208493818738, 76.10064029115018513 ) ) ;
#9531=DIRECTION ( 'NONE',  ( 0.000000000000000000, -0.000000000000000000, 1.000000000000000000 ) ) ;
#9540=EDGE_LOOP ( 'NONE', ( #4637, #4046, #14578, #9361, #3740, #9309, #11836, #11645, #13152, #3055 ) ) ;
#9543=ORIENTED_EDGE ( 'NONE', *, *, #6195, .F. ) ;
#9549=ORIENTED_EDGE ( 'NONE', *, *, #10598, .T. ) ;
#9550=CIRCLE ( 'NONE', #6823, 0.7892041907098261699 ) ;
#9553=CARTESIAN_POINT ( 'NONE',  ( 60.34603303165619792, -7.282908750500069139, 54.56811043785583593 ) ) ;
#9555=CARTESIAN_POINT ( 'NONE',  ( 4.848008884920353090, 21.49656883983473676, 75.19766410831374515 ) ) ;
#9556=CARTESIAN_POINT ( 'NONE',  ( 70.26445833701072274, -4.474174595298148205, 72.19766410831374515 ) ) ;
#9566=ORIENTED_EDGE ( 'NONE', *, *, #706, .T. ) ;
#9577=AXIS2_PLACEMENT_3D ( 'NONE', #12081, #6090, #8611 ) ;
#9583=ADVANCED_FACE ( 'NONE', ( #14102 ), #3554, .T. ) ;
#9588=ORIENTED_EDGE ( 'NONE', *, *, #14373, .T. ) ;
#9590=CARTESIAN_POINT ( 'NONE',  ( 119.1667258010536301, -36.15456035933797807, 56.28371344025897827 ) ) ;
#9600=ORIENTED_EDGE ( 'NONE', *, *, #10206, .T. ) ;
#9604=CARTESIAN_POINT ( 'NONE',  ( 64.11356538205144773, -11.94785243701160127, 75.33582547088241199 ) ) ;
#9607=FACE_OUTER_BOUND ( 'NONE', #12392, .T. ) ;
#9611=AXIS2_PLACEMENT_3D ( 'NONE', #8740, #3127, #6588 ) ;
#9615=VERTEX_POINT ( 'NONE', #7751 ) ;
#9617=ORIENTED_EDGE ( 'NONE', *, *, #14583, .F. ) ;
#9619=VERTEX_POINT ( 'NONE', #12007 ) ;
#9621=EDGE_LOOP ( 'NONE', ( #3157, #11702, #13429, #10208 ) ) ;
#9624=EDGE_LOOP ( 'NONE', ( #7845, #12078, #7755, #8336 ) ) ;
#9628=EDGE_CURVE ( 'NONE', #5320, #8533, #14640, .T. ) ;
#9631=CARTESIAN_POINT ( 'NONE',  ( 69.99947051259638897, -3.232128232595322448, 72.90093656932181432 ) ) ;
#9639=ORIENTED_EDGE ( 'NONE', *, *, #13649, .T. ) ;
#9640=DIRECTION ( 'NONE',  ( -1.224646799147353207E-16, 1.000000000000000000, 0.000000000000000000 ) ) ;
#9643=VECTOR ( 'NONE', #4383, 1000.000000000000000 ) ;
#9648=PRODUCT_CONTEXT ( 'NONE', #11879, 'mechanical' ) ;
#9662=DIRECTION ( 'NONE',  ( -0.000000000000000000, 0.000000000000000000, -1.000000000000000000 ) ) ;
#9667=CARTESIAN_POINT ( 'NONE',  ( 118.2606911748681568, -35.65233716510192608, 53.46824312087640863 ) ) ;
#9671=CARTESIAN_POINT ( 'NONE',  ( 64.34486446596575604, -11.79842398862770736, 72.19615287623349786 ) ) ;
#9674=CARTESIAN_POINT ( 'NONE',  ( 70.22985855910454234, -4.172664678593861254, 76.17430469024502315 ) ) ;
#9679=AXIS2_PLACEMENT_3D ( 'NONE', #12301, #1756, #1128 ) ;
#9680=DIRECTION ( 'NONE',  ( 0.000000000000000000, 0.000000000000000000, 1.000000000000000000 ) ) ;
#9682=CIRCLE ( 'NONE', #11626, 1.000000000000000888 ) ;
#9692=EDGE_CURVE ( 'NONE', #11155, #2180, #9125, .T. ) ;
#9694=AXIS2_PLACEMENT_3D ( 'NONE', #9908, #14587, #4036 ) ;
#9708=VERTEX_POINT ( 'NONE', #3059 ) ;
#9712=VERTEX_POINT ( 'NONE', #11274 ) ;
#9714=DIRECTION ( 'NONE',  ( 0.7398406760702315177, 0.6727821148276332819, 8.214872995831076759E-16 ) ) ;
#9715=B_SPLINE_CURVE_WITH_KNOTS ( 'NONE', 3,
 ( #6253, #1313, #6312, #13021, #4932, #7394, #11007, #11926, #2697, #14474 ),
 .UNSPECIFIED., .F., .F.,
 ( 4, 2, 2, 2, 4 ),
 ( 0.000000000000000000, 0.0004605959310618659556, 0.0009211918621237319112, 0.001381787793185597921, 0.001842383724247463822 ),
 .UNSPECIFIED. ) ;
#9720=EDGE_CURVE ( 'NONE', #3629, #14995, #1633, .T. ) ;
#9721=EDGE_LOOP ( 'NONE', ( #5944, #2533, #739, #5769 ) ) ;
#9722=DIRECTION ( 'NONE',  ( 0.8746197071345573892, -0.4848096202550657430, 0.000000000000000000 ) ) ;
#9725=DIRECTION ( 'NONE',  ( -0.3020115420618222357, 0.1674077314120182292, -0.9384901064608630605 ) ) ;
#9728=FACE_OUTER_BOUND ( 'NONE', #5370, .T. ) ;
#9731=DIRECTION ( 'NONE',  ( -0.000000000000000000, 0.000000000000000000, -1.000000000000000000 ) ) ;
#9742=CARTESIAN_POINT ( 'NONE',  ( 76.63070922904937277, -6.859691020777845871, 75.19766410831374515 ) ) ;
#9748=CARTESIAN_POINT ( 'NONE',  ( 58.00000000000000711, -2.249290599286311032, -38.00000000000012079 ) ) ;
#9764=AXIS2_PLACEMENT_3D ( 'NONE', #6300, #8678, #10846 ) ;
#9767=CARTESIAN_POINT ( 'NONE',  ( 64.16994054879148734, -11.91212264076314575, 75.71502901994244894 ) ) ;
#9770=EDGE_LOOP ( 'NONE', ( #2908, #13650, #9147, #2247, #14740, #8614, #4298 ) ) ;
#9782=FACE_OUTER_BOUND ( 'NONE', #13588, .T. ) ;
#9784=CIRCLE ( 'NONE', #4867, 0.9999999999999957812 ) ;
#9786=ORIENTED_EDGE ( 'NONE', *, *, #4897, .F. ) ;
#9789=ORIENTED_EDGE ( 'NONE', *, *, #12920, .F. ) ;
#9790=CIRCLE ( 'NONE', #13459, 1.000000000000000888 ) ;
#9795=FACE_OUTER_BOUND ( 'NONE', #8873, .T. ) ;
#9801=ADVANCED_FACE ( 'NONE', ( #4672 ), #159, .T. ) ;
#9810=EDGE_CURVE ( 'NONE', #12141, #14247, #11957, .T. ) ;
#9812=ORIENTED_EDGE ( 'NONE', *, *, #242, .F. ) ;
#9817=CARTESIAN_POINT ( 'NONE',  ( 64.12538157620423362, -11.94043129933760206, 72.93296134066703473 ) ) ;
#9828=CARTESIAN_POINT ( 'NONE',  ( 63.36453054171181520, -0.8129776999179910701, 60.61639468829817190 ) ) ;
#9844=CYLINDRICAL_SURFACE ( 'NONE', #2977, 0.7892041907098261699 ) ;
#9847=VERTEX_POINT ( 'NONE', #137 ) ;
#9849=DIRECTION ( 'NONE',  ( 0.000000000000000000, 0.000000000000000000, 1.000000000000000000 ) ) ;
#9857=ADVANCED_FACE ( 'NONE', ( #5052 ), #8299, .T. ) ;
#9865=LINE ( 'NONE', #12006, #7927 ) ;
#9866=AXIS2_PLACEMENT_3D ( 'NONE', #10764, #5928, #4835 ) ;
#9871=VECTOR ( 'NONE', #1348, 1000.000000000000000 ) ;
#9874=DIRECTION ( 'NONE',  ( 0.7392394270158823000, -0.6734426995262700055, 0.000000000000000000 ) ) ;
#9877=CIRCLE ( 'NONE', #4952, 0.7892041907098278353 ) ;
#9881=DIRECTION ( 'NONE',  ( -0.8746197071345571672, 0.4848096202550660205, 0.000000000000000000 ) ) ;
#9887=CIRCLE ( 'NONE', #3241, 0.7892041907098262810 ) ;
#9893=CIRCLE ( 'NONE', #5975, 3.999999999999994227 ) ;
#9894=ORIENTED_EDGE ( 'NONE', *, *, #4862, .T. ) ;
#9895=EDGE_CURVE ( 'NONE', #14607, #6894, #12206, .T. ) ;
#9899=EDGE_CURVE ( 'NONE', #6894, #14607, #2865, .T. ) ;
#9906=CARTESIAN_POINT ( 'NONE',  ( 33.53865989972762662, 5.593081289880174722, 89.15517579724127017 ) ) ;
#9908=CARTESIAN_POINT ( 'NONE',  ( 72.26742264675378635, -14.73126838498886571, 75.19766410831374515 ) ) ;
#9915=( BOUNDED_SURFACE ( )  B_SPLINE_SURFACE ( 3, 2, ( 
 ( #5914, #5994, #8298 ),
 ( #9604, #2518, #13136 ),
 ( #136, #4671, #2439 ),
 ( #3739, #6139, #1207 ),
 ( #10596, #6983, #14371 ),
 ( #10824, #283, #7135 ),
 ( #12840, #7281, #2289 ),
 ( #11899, #12918, #61 ),
 ( #4978, #9370, #4823 ),
 ( #4754, #8225, #9450 ),
 ( #2362, #14142, #9528 ),
 ( #3590, #14218, #6059 ),
 ( #3669, #8371, #13062 ),
 ( #1358, #10751, #11969 ) ),
 .UNSPECIFIED., .F., .F., .F. ) 
 B_SPLINE_SURFACE_WITH_KNOTS ( ( 4, 2, 2, 2, 2, 2, 4 ),
 ( 3, 3 ),
 ( 0.001231944704344891230, 0.001640530120327067607, 0.002049115536309244201, 0.002866286368273596955, 0.003274871784255773549, 0.003683457200237949709, 0.004500628032202302897 ),
 ( 0.000000000000000000, 1.000000000000000000 ),
 .UNSPECIFIED. ) 
 GEOMETRIC_REPRESENTATION_ITEM ( )  RATIONAL_B_SPLINE_SURFACE ( (
 ( 1.000000000000000000, 0.8606282562001377201, 1.000000000000000000),
 ( 1.000000000000000000, 0.8606242962982729727, 1.000000000000000000),
 ( 1.000000000000000000, 0.8593044206444694355, 1.000000000000000000),
 ( 1.000000000000000000, 0.8542070032136860336, 1.000000000000000000),
 ( 1.000000000000000000, 0.8503651661365319026, 1.000000000000000000),
 ( 1.000000000000000000, 0.8359148296419828261, 1.000000000000000000),
 ( 1.000000000000000000, 0.8221039232031693844, 1.000000000000000000),
 ( 1.000000000000000000, 0.7986554744404532613, 1.000000000000000000),
 ( 1.000000000000000000, 0.7902603328757243917, 1.000000000000000000),
 ( 1.000000000000000000, 0.7732499594492155959, 1.000000000000000000),
 ( 1.000000000000000000, 0.7646145331269290635, 1.000000000000000000),
 ( 1.000000000000000000, 0.7387090984033097829, 1.000000000000000000),
 ( 1.000000000000000000, 0.7216377403000998614, 1.000000000000000000),
 ( 1.000000000000000000, 0.7071067811865457964, 1.000000000000000000) ) ) 
 REPRESENTATION_ITEM ( '' )  SURFACE ( )  );
#9929=CARTESIAN_POINT ( 'NONE',  ( 63.04142083571589694, -2.691337429055927988, 62.84860122826521689 ) ) ;
#9930=DIRECTION ( 'NONE',  ( -0.8746197071345572782, 0.4848096202550659650, 0.000000000000000000 ) ) ;
#9931=DIRECTION ( 'NONE',  ( -1.000000000000000000, 0.000000000000000000, 0.000000000000000000 ) ) ;
#9932=ORIENTED_EDGE ( 'NONE', *, *, #8499, .F. ) ;
#9935=CIRCLE ( 'NONE', #7475, 0.7892041907098261699 ) ;
#9940=DIRECTION ( 'NONE',  ( 0.000000000000000000, -3.469446951953611033E-15, 1.000000000000000000 ) ) ;
#9942=ADVANCED_FACE ( 'NONE', ( #9607 ), #6072, .T. ) ;
#9946=DIRECTION ( 'NONE',  ( -0.000000000000000000, -0.000000000000000000, 1.000000000000000000 ) ) ;
#9958=ORIENTED_EDGE ( 'NONE', *, *, #9193, .F. ) ;
#9959=DIRECTION ( 'NONE',  ( 0.3020115420618248447, -0.1674077314120183957, 0.9384901064608620613 ) ) ;
#9961=DIRECTION ( 'NONE',  ( -0.000000000000000000, -0.000000000000000000, 1.000000000000000000 ) ) ;
#9965=ORIENTED_EDGE ( 'NONE', *, *, #13939, .F. ) ;
#9971=EDGE_CURVE ( 'NONE', #9847, #12140, #3615, .T. ) ;
#9973=ADVANCED_FACE ( 'NONE', ( #1436 ), #14444, .T. ) ;
#9985=AXIS2_PLACEMENT_3D ( 'NONE', #12601, #3361, #7905 ) ;
#10005=DIRECTION ( 'NONE',  ( -0.000000000000000000, -0.000000000000000000, -1.000000000000000000 ) ) ;
#10011=CIRCLE ( 'NONE', #14669, 0.9999999999999960032 ) ;
#10013=CARTESIAN_POINT ( 'NONE',  ( 70.14667088542560691, -3.748710008331756605, 76.02364810721972788 ) ) ;
#10014=DIRECTION ( 'NONE',  ( 0.000000000000000000, 0.000000000000000000, 1.000000000000000000 ) ) ;
#10023=CARTESIAN_POINT ( 'NONE',  ( 58.00000000000000711, -2.249290599286309256, 77.19766410831374515 ) ) ;
#10030=DIRECTION ( 'NONE',  ( -0.8746197071345572782, 0.4848096202550659650, -0.000000000000000000 ) ) ;
#10034=CIRCLE ( 'NONE', #5363, 0.7892041907098277242 ) ;
#10047=CARTESIAN_POINT ( 'NONE',  ( 121.5439789431140554, -37.47229329360762762, 52.08701862022444118 ) ) ;
#10048=FACE_OUTER_BOUND ( 'NONE', #3265, .T. ) ;
#10056=AXIS2_PLACEMENT_3D ( 'NONE', #15188, #1179, #8345 ) ;
#10068=AXIS2_PLACEMENT_3D ( 'NONE', #7988, #7497, #7065 ) ;
#10070=CIRCLE ( 'NONE', #10813, 1.000000000000000888 ) ;
#10078=ORIENTED_EDGE ( 'NONE', *, *, #15154, .T. ) ;
#10080=DIRECTION ( 'NONE',  ( 0.8746197071345571672, -0.4848096202550660205, 0.000000000000000000 ) ) ;
#10085=LINE ( 'NONE', #11229, #3829 ) ;
#10087=DIRECTION ( 'NONE',  ( 0.000000000000000000, 0.000000000000000000, 1.000000000000000000 ) ) ;
#10088=CARTESIAN_POINT ( 'NONE',  ( 65.49059688361914766, -11.82389893047565543, 72.52483798894591871 ) ) ;
#10089=CARTESIAN_POINT ( 'NONE',  ( 69.36198185152332485, -3.785319131685315419, 77.13117128918304388 ) ) ;
#10109=CYLINDRICAL_SURFACE ( 'NONE', #1266, 0.7892041907098262810 ) ;
#10113=ORIENTED_EDGE ( 'NONE', *, *, #14320, .T. ) ;
#10121=AXIS2_PLACEMENT_3D ( 'NONE', #3, #4926, #4694 ) ;
#10123=EDGE_CURVE ( 'NONE', #13525, #13763, #6321, .T. ) ;
#10124=B_SPLINE_CURVE_WITH_KNOTS ( 'NONE', 3,
 ( #2655, #11303, #9674, #8769, #10013, #6127, #10814, #762, #5475, #10165 ),
 .UNSPECIFIED., .F., .F.,
 ( 4, 2, 2, 2, 4 ),
 ( 0.000000000000000000, 0.0004549325576484883273, 0.0009098651152969778472, 0.001364797672945467421, 0.001819730230593956995 ),
 .UNSPECIFIED. ) ;
#10131=DIRECTION ( 'NONE',  ( -0.8746197071345569451, 0.4848096202550666312, 0.000000000000000000 ) ) ;
#10134=EDGE_LOOP ( 'NONE', ( #8379, #3482, #5261, #147 ) ) ;
#10144=CARTESIAN_POINT ( 'NONE',  ( 58.00000000000000711, -2.249290599286309256, 38.50000000000012790 ) ) ;
#10146=CARTESIAN_POINT ( 'NONE',  ( 65.46376463298187787, -11.83285265143084963, 75.85541229843748567 ) ) ;
#10148=CARTESIAN_POINT ( 'NONE',  ( 52.94134894379979528, -2.395505968190773327, 48.51982618741349285 ) ) ;
#10154=CARTESIAN_POINT ( 'NONE',  ( 76.78650653802468184, -6.946050879336882922, 76.19766410831374515 ) ) ;
#10163=VERTEX_POINT ( 'NONE', #873 ) ;
#10165=CARTESIAN_POINT ( 'NONE',  ( 69.97972559857382180, -3.172990593254279457, 75.19766410831374515 ) ) ;
#10172=ORIENTED_EDGE ( 'NONE', *, *, #10928, .F. ) ;
#10181=DIRECTION ( 'NONE',  ( -0.000000000000000000, 0.000000000000000000, -1.000000000000000000 ) ) ;
#10191=EDGE_CURVE ( 'NONE', #14840, #1587, #2106, .T. ) ;
#10202=CARTESIAN_POINT ( 'NONE',  ( 62.14609464170151654, 0.6526447315840442354, 60.61639468829817190 ) ) ;
#10206=EDGE_CURVE ( 'NONE', #13687, #7654, #8040, .T. ) ;
#10208=ORIENTED_EDGE ( 'NONE', *, *, #667, .F. ) ;
#10220=DIRECTION ( 'NONE',  ( -0.8746197071345558349, 0.4848096202550685185, 0.000000000000000000 ) ) ;
#10223=EDGE_CURVE ( 'NONE', #3495, #14121, #14662, .T. ) ;
#10224=CIRCLE ( 'NONE', #13401, 1.000000000000000888 ) ;
#10230=CARTESIAN_POINT ( 'NONE',  ( 68.90181265608016759, -8.292264031936127822, 71.19766410831374515 ) ) ;
#10232=CIRCLE ( 'NONE', #6542, 0.7892041907098262810 ) ;
#10237=CARTESIAN_POINT ( 'NONE',  ( 64.61411691182244965, -11.63232581036083069, 73.19766410831374515 ) ) ;
#10238=CARTESIAN_POINT ( 'NONE',  ( 69.43429300475483501, -3.089800330891553148, 76.78179314627131191 ) ) ;
#10244=CIRCLE ( 'NONE', #12960, 1.000000000000000888 ) ;
#10245=AXIS2_PLACEMENT_3D ( 'NONE', #4755, #213, #7209 ) ;
#10250=LINE ( 'NONE', #12404, #11045 ) ;
#10259=AXIS2_PLACEMENT_3D ( 'NONE', #5175, #4083, #9881 ) ;
#10260=FACE_OUTER_BOUND ( 'NONE', #13413, .T. ) ;
#10263=ADVANCED_FACE ( 'NONE', ( #4574 ), #4652, .T. ) ;
#10264=DIRECTION ( 'NONE',  ( 0.000000000000000000, 0.000000000000000000, 1.000000000000000000 ) ) ;
#10265=VERTEX_POINT ( 'NONE', #13969 ) ;
#10274=AXIS2_PLACEMENT_3D ( 'NONE', #4065, #13387, #12096 ) ;
#10285=CIRCLE ( 'NONE', #14221, 0.7892041907098262810 ) ;
#10300=CARTESIAN_POINT ( 'NONE',  ( 66.38598137497019991, -11.47113225237460910, 76.19766410831374515 ) ) ;
#10304=ORIENTED_EDGE ( 'NONE', *, *, #7447, .T. ) ;
#10308=ORIENTED_EDGE ( 'NONE', *, *, #10722, .T. ) ;
#10314=ADVANCED_FACE ( 'NONE', ( #14356 ), #13122, .T. ) ;
#10315=ORIENTED_EDGE ( 'NONE', *, *, #1043, .T. ) ;
#10318=DIRECTION ( 'NONE',  ( 0.000000000000000000, 0.000000000000000000, 1.000000000000000000 ) ) ;
#10323=CARTESIAN_POINT ( 'NONE',  ( 69.43190845037254633, -3.121612608933937327, 71.58974242810022304 ) ) ;
#10324=CIRCLE ( 'NONE', #6387, 11.46463184759104692 ) ;
#10339=DIRECTION ( 'NONE',  ( 0.7915791710638007128, 0.6110666215217015473, 0.000000000000000000 ) ) ;
#10340=EDGE_LOOP ( 'NONE', ( #6083, #2857, #1103, #13445 ) ) ;
#10343=ORIENTED_EDGE ( 'NONE', *, *, #10547, .F. ) ;
#10363=AXIS2_PLACEMENT_3D ( 'NONE', #12866, #3766, #2384 ) ;
#10371=DIRECTION ( 'NONE',  ( -0.000000000000000000, 0.000000000000000000, -1.000000000000000000 ) ) ;
#10375=AXIS2_PLACEMENT_3D ( 'NONE', #9396, #14393, #1459 ) ;
#10376=CARTESIAN_POINT ( 'NONE',  ( 65.14440678340884006, -11.91619605160587803, 75.34954452637725808 ) ) ;
#10386=CIRCLE ( 'NONE', #10629, 8.924024642120691908 ) ;
#10402=ORIENTED_EDGE ( 'NONE', *, *, #11023, .T. ) ;
#10404=CARTESIAN_POINT ( 'NONE',  ( 69.30279253104961867, -4.172890756685618818, 72.15742259932318348 ) ) ;
#10407=EDGE_CURVE ( 'NONE', #4043, #13455, #1406, .T. ) ;
#10419=CARTESIAN_POINT ( 'NONE',  ( 75.52271037289314393, -7.388871293676331220, 73.19766410831374515 ) ) ;
#10420=EDGE_CURVE ( 'NONE', #3522, #8564, #2640, .T. ) ;
#10424=ORIENTED_EDGE ( 'NONE', *, *, #12393, .T. ) ;
#10427=EDGE_LOOP ( 'NONE', ( #4448, #6281, #4884, #5571 ) ) ;
#10441=ORIENTED_EDGE ( 'NONE', *, *, #740, .T. ) ;
#10449=EDGE_CURVE ( 'NONE', #2182, #5691, #3368, .T. ) ;
#10450=EDGE_CURVE ( 'NONE', #3036, #14454, #12028, .T. ) ;
#10462=ORIENTED_EDGE ( 'NONE', *, *, #196, .T. ) ;
#10466=EDGE_CURVE ( 'NONE', #10163, #13455, #1260, .T. ) ;
#10467=CARTESIAN_POINT ( 'NONE',  ( 76.93272077111119245, -7.027098752189868236, 76.13615421477460643 ) ) ;
#10472=DIRECTION ( 'NONE',  ( 0.000000000000000000, 0.000000000000000000, 1.000000000000000000 ) ) ;
#10473=ADVANCED_FACE ( 'NONE', ( #12256 ), #4015, .T. ) ;
#10477=CARTESIAN_POINT ( 'NONE',  ( 70.12227446635188244, -3.653170910121650738, 72.43426084522523922 ) ) ;
#10478=ORIENTED_EDGE ( 'NONE', *, *, #1656, .F. ) ;
#10479=LINE ( 'NONE', #11780, #3501 ) ;
#10484=VERTEX_POINT ( 'NONE', #6404 ) ;
#10485=EDGE_CURVE ( 'NONE', #11588, #4043, #11173, .T. ) ;
#10486=FACE_OUTER_BOUND ( 'NONE', #8101, .T. ) ;
#10491=EDGE_CURVE ( 'NONE', #3380, #9847, #15172, .T. ) ;
#10497=EDGE_LOOP ( 'NONE', ( #8155, #9196, #13575, #7095 ) ) ;
#10498=CARTESIAN_POINT ( 'NONE',  ( 50.07597535787931520, -2.249290599286309256, 47.51982618741348574 ) ) ;
#10506=CARTESIAN_POINT ( 'NONE',  ( 54.03086304124234829, 0.8903401505190762233, 48.51982618741349285 ) ) ;
#10509=EDGE_CURVE ( 'NONE', #384, #1157, #3861, .T. ) ;
#10511=CYLINDRICAL_SURFACE ( 'NONE', #11975, 0.7892041907098261699 ) ;
#10518=ORIENTED_EDGE ( 'NONE', *, *, #3436, .T. ) ;
#10519=AXIS2_PLACEMENT_3D ( 'NONE', #6629, #1087, #2245 ) ;
#10521=VERTEX_POINT ( 'NONE', #7561 ) ;
#10526=DIRECTION ( 'NONE',  ( -0.000000000000000000, -0.000000000000000000, -1.000000000000000000 ) ) ;
#10534=CARTESIAN_POINT ( 'NONE',  ( 72.26742264675378635, -14.73126838498886571, 75.19766410831374515 ) ) ;
#10542=ORIENTED_EDGE ( 'NONE', *, *, #4364, .F. ) ;
#10543=EDGE_CURVE ( 'NONE', #14082, #9158, #3122, .T. ) ;
#10545=DIRECTION ( 'NONE',  ( 0.000000000000000000, 0.000000000000000000, -1.000000000000000000 ) ) ;
#10547=EDGE_CURVE ( 'NONE', #12099, #12141, #4347, .T. ) ;
#10558=EDGE_CURVE ( 'NONE', #11155, #6181, #3627, .T. ) ;
#10561=AXIS2_PLACEMENT_3D ( 'NONE', #3791, #5317, #14345 ) ;
#10568=ORIENTED_EDGE ( 'NONE', *, *, #13345, .T. ) ;
#10575=CIRCLE ( 'NONE', #3439, 0.7892041907098262810 ) ;
#10576=CARTESIAN_POINT ( 'NONE',  ( 119.1667258010536301, -36.15456035933797807, 56.28371344025898537 ) ) ;
#10578=DIRECTION ( 'NONE',  ( -0.4848096202550659650, -0.8746197071345573892, 0.000000000000000000 ) ) ;
#10583=DIRECTION ( 'NONE',  ( -0.3255681544665827709, -0.9455185755960711091, 0.000000000000000000 ) ) ;
#10591=CARTESIAN_POINT ( 'NONE',  ( 54.86190032082818391, 1.721056973166403603, 62.84860122826521689 ) ) ;
#10594=ORIENTED_EDGE ( 'NONE', *, *, #4382, .T. ) ;
#10596=CARTESIAN_POINT ( 'NONE',  ( 64.21144059111647096, -11.88561900177543329, 75.86747644619509856 ) ) ;
#10598=EDGE_CURVE ( 'NONE', #6506, #14878, #5594, .T. ) ;
#10607=ORIENTED_EDGE ( 'NONE', *, *, #15217, .F. ) ;
#10610=CARTESIAN_POINT ( 'NONE',  ( 64.77146624638496064, -11.50114768494419160, 76.78128728924484392 ) ) ;
#10620=CIRCLE ( 'NONE', #12836, 0.7892041907098290565 ) ;
#10629=AXIS2_PLACEMENT_3D ( 'NONE', #679, #12541, #11591 ) ;
#10630=CYLINDRICAL_SURFACE ( 'NONE', #11245, 0.9999999999999954481 ) ;
#10632=AXIS2_PLACEMENT_3D ( 'NONE', #12011, #2706, #2784 ) ;
#10635=DIRECTION ( 'NONE',  ( -0.000000000000000000, 0.000000000000000000, -1.000000000000000000 ) ) ;
#10636=DIRECTION ( 'NONE',  ( 0.000000000000000000, 0.000000000000000000, 1.000000000000000000 ) ) ;
#10639=ADVANCED_FACE ( 'NONE', ( #3871 ), #408, .T. ) ;
#10646=EDGE_CURVE ( 'NONE', #11917, #879, #13633, .T. ) ;
#10651=CARTESIAN_POINT ( 'NONE',  ( 63.04142083571589694, -2.691337429055927988, 60.61639468829817190 ) ) ;
#10653=EDGE_CURVE ( 'NONE', #11350, #14454, #5860, .T. ) ;
#10661=DIRECTION ( 'NONE',  ( 0.3020115420618265656, -0.1674077314120193949, 0.9384901064608611732 ) ) ;
#10663=CARTESIAN_POINT ( 'NONE',  ( 70.08913995591909440, -3.527907623570947226, 75.87049022768096052 ) ) ;
#10666=LINE ( 'NONE', #8212, #2489 ) ;
#10670=AXIS2_PLACEMENT_3D ( 'NONE', #4048, #306, #2609 ) ;
#10672=FACE_OUTER_BOUND ( 'NONE', #2059, .T. ) ;
#10680=LINE ( 'NONE', #2441, #1303 ) ;
#10684=EDGE_CURVE ( 'NONE', #13307, #5064, #1416, .T. ) ;
#10700=ORIENTED_EDGE ( 'NONE', *, *, #9079, .T. ) ;
#10708=CARTESIAN_POINT ( 'NONE',  ( 65.92402464212069901, -2.249290599286309256, 38.50000000000012790 ) ) ;
#10710=CARTESIAN_POINT ( 'NONE',  ( 58.00000000000000711, -2.249290599286309256, 71.19766410831374515 ) ) ;
#10722=EDGE_CURVE ( 'NONE', #8760, #9351, #4872, .T. ) ;
#10725=DIRECTION ( 'NONE',  ( -0.000000000000000000, -1.000000000000000000, -0.000000000000000000 ) ) ;
#10732=CARTESIAN_POINT ( 'NONE',  ( 64.94561305207867008, -11.37113100889128248, 71.46833336701176620 ) ) ;
#10733=EDGE_CURVE ( 'NONE', #7249, #14177, #9790, .T. ) ;
#10749=AXIS2_PLACEMENT_3D ( 'NONE', #12656, #3271, #13887 ) ;
#10751=CARTESIAN_POINT ( 'NONE',  ( 65.71319926014257362, -10.73129157630437014, 76.19766410831375936 ) ) ;
#10752=DIRECTION ( 'NONE',  ( -1.000000000000000000, 0.000000000000000000, 0.000000000000000000 ) ) ;
#10759=DIRECTION ( 'NONE',  ( 0.8746197071345560570, -0.4848096202550682410, 0.000000000000000000 ) ) ;
#10763=EDGE_LOOP ( 'NONE', ( #11294, #14751 ) ) ;
#10764=CARTESIAN_POINT ( 'NONE',  ( 58.00000000000000711, -2.249290599286309256, 86.40005259842790508 ) ) ;
#10768=ORIENTED_EDGE ( 'NONE', *, *, #11339, .T. ) ;
#10772=CARTESIAN_POINT ( 'NONE',  ( 69.44738493598792672, -2.877909345519603868, 73.19766410831374515 ) ) ;
#10774=EDGE_CURVE ( 'NONE', #6522, #7200, #6825, .T. ) ;
#10779=TOROIDAL_SURFACE ( 'NONE', #6115, 3.999999999999996447, 1.000000000000000000 ) ;
#10786=EDGE_LOOP ( 'NONE', ( #2646, #13842, #4216, #8553 ) ) ;
#10795=PLANE ( 'NONE',  #11192 ) ;
#10813=AXIS2_PLACEMENT_3D ( 'NONE', #10498, #10725, #2572 ) ;
#10814=CARTESIAN_POINT ( 'NONE',  ( 70.05014002589594213, -3.391651902948124242, 75.75351273523833129 ) ) ;
#10815=DIRECTION ( 'NONE',  ( 0.000000000000000000, 0.000000000000000000, -1.000000000000000000 ) ) ;
#10824=CARTESIAN_POINT ( 'NONE',  ( 64.34994344588844228, -11.79539688520061702, 76.23544073996576742 ) ) ;
#10831=CIRCLE ( 'NONE', #14749, 0.7892041907098262810 ) ;
#10834=FACE_OUTER_BOUND ( 'NONE', #6022, .T. ) ;
#10839=ADVANCED_FACE ( 'NONE', ( #11785 ), #2561, .T. ) ;
#10842=ORIENTED_EDGE ( 'NONE', *, *, #15217, .T. ) ;
#10843=CARTESIAN_POINT ( 'NONE',  ( 56.97758043373130477, 2.707118148285912795, 48.51982618741349285 ) ) ;
#10846=DIRECTION ( 'NONE',  ( -0.3020115420618285085, 0.1674077314120178406, -0.9384901064608609511 ) ) ;
#10854=CIRCLE ( 'NONE', #760, 0.7892041907098278353 ) ;
#10866=CARTESIAN_POINT ( 'NONE',  ( 69.28051765693513175, -4.295678830383772961, 71.19766410831374515 ) ) ;
#10871=CARTESIAN_POINT ( 'NONE',  ( 9.696105087471012851, 30.24276591118031021, 0.000000000000000000 ) ) ;
#10877=FACE_OUTER_BOUND ( 'NONE', #5728, .T. ) ;
#10882=ADVANCED_FACE ( 'NONE', ( #13172 ), #2628, .T. ) ;
#10891=CARTESIAN_POINT ( 'NONE',  ( 69.39844472759932614, -3.556430582623343550, 76.16265406106171554 ) ) ;
#10893=CARTESIAN_POINT ( 'NONE',  ( 65.43388225677183812, -11.84036758951991963, 72.57413203708259175 ) ) ;
#10896=ADVANCED_FACE ( 'NONE', ( #9795 ), #438, .F. ) ;
#10897=EDGE_CURVE ( 'NONE', #11609, #6596, #9286, .T. ) ;
#10898=CARTESIAN_POINT ( 'NONE',  ( 70.04068982727432058, -3.360887980114144025, 72.67877579342776073 ) ) ;
#10900=CIRCLE ( 'NONE', #12619, 0.7892041907098262810 ) ;
#10909=DIRECTION ( 'NONE',  ( 0.000000000000000000, 0.000000000000000000, 1.000000000000000000 ) ) ;
#10912=VERTEX_POINT ( 'NONE', #8621 ) ;
#10913=AXIS2_PLACEMENT_3D ( 'NONE', #10202, #13508, #12589 ) ;
#10919=DIRECTION ( 'NONE',  ( -0.8746197071345572782, 0.4848096202550659650, 0.000000000000000000 ) ) ;
#10928=EDGE_CURVE ( 'NONE', #1582, #153, #11977, .T. ) ;
#10941=ADVANCED_FACE ( 'NONE', ( #2783 ), #2844, .T. ) ;
#10943=EDGE_CURVE ( 'NONE', #943, #3036, #6098, .T. ) ;
#10944=CARTESIAN_POINT ( 'NONE',  ( 116.6234642359097222, -39.31822372505217089, 54.40673322733726991 ) ) ;
#10945=ORIENTED_EDGE ( 'NONE', *, *, #1603, .T. ) ;
#10959=DIRECTION ( 'NONE',  ( -0.000000000000000000, -0.000000000000000000, -1.000000000000000000 ) ) ;
#10967=ORIENTED_EDGE ( 'NONE', *, *, #11473, .T. ) ;
#10973=CARTESIAN_POINT ( 'NONE',  ( 54.07385127050791596, 1.678372679529495981, 60.61639468829817190 ) ) ;
#10975=ADVANCED_FACE ( 'NONE', ( #1623 ), #327, .T. ) ;
#10977=EDGE_CURVE ( 'NONE', #7233, #3522, #8053, .T. ) ;
#10980=VERTEX_POINT ( 'NONE', #833 ) ;
#10992=AXIS2_PLACEMENT_3D ( 'NONE', #8366, #7046, #7129 ) ;
#11001=DIRECTION ( 'NONE',  ( -0.000000000000000000, 0.000000000000000000, -1.000000000000000000 ) ) ;
#11007=CARTESIAN_POINT ( 'NONE',  ( 65.83943508202165162, -11.71002111017040193, 72.30872443868064181 ) ) ;
#11023=EDGE_CURVE ( 'NONE', #5064, #6181, #12235, .T. ) ;
#11025=EDGE_CURVE ( 'NONE', #9619, #10912, #7564, .T. ) ;
#11040=EDGE_LOOP ( 'NONE', ( #6997, #2340, #4117, #7914 ) ) ;
#11041=DIRECTION ( 'NONE',  ( -0.000000000000000000, 0.000000000000000000, -1.000000000000000000 ) ) ;
#11042=ORIENTED_EDGE ( 'NONE', *, *, #14497, .F. ) ;
#11045=VECTOR ( 'NONE', #4473, 1000.000000000000000 ) ;
#11055=DIRECTION ( 'NONE',  ( -0.8746197071345570562, 0.4848096202550665756, 0.000000000000000000 ) ) ;
#11071=DIRECTION ( 'NONE',  ( 0.2135987722749887463, 0.9769214730379394140, 0.000000000000000000 ) ) ;
#11072=VERTEX_POINT ( 'NONE', #2070 ) ;
#11078=CARTESIAN_POINT ( 'NONE',  ( 59.59091026602544616, -7.053490217115945704, 48.51982618741349285 ) ) ;
#11088=CIRCLE ( 'NONE', #12324, 0.7892041907098291675 ) ;
#11092=EDGE_CURVE ( 'NONE', #931, #879, #885, .T. ) ;
#11096=DIRECTION ( 'NONE',  ( 1.000000000000000000, 0.000000000000000000, 0.000000000000000000 ) ) ;
#11097=DIRECTION ( 'NONE',  ( -0.000000000000000000, 0.000000000000000000, -1.000000000000000000 ) ) ;
#11099=EDGE_CURVE ( 'NONE', #1157, #6894, #13196, .T. ) ;
#11101=FACE_OUTER_BOUND ( 'NONE', #8081, .T. ) ;
#11105=AXIS2_PLACEMENT_3D ( 'NONE', #7995, #1065, #5619 ) ;
#11118=ORIENTED_EDGE ( 'NONE', *, *, #14553, .T. ) ;
#11119=DIRECTION ( 'NONE',  ( 0.8746197071345569451, -0.4848096202550666312, 0.000000000000000000 ) ) ;
#11130=ORIENTED_EDGE ( 'NONE', *, *, #4617, .F. ) ;
#11140=LINE ( 'NONE', #6241, #2802 ) ;
#11147=LINE ( 'NONE', #7609, #423 ) ;
#11155=VERTEX_POINT ( 'NONE', #6081 ) ;
#11157=DIRECTION ( 'NONE',  ( 0.000000000000000000, 0.000000000000000000, 1.000000000000000000 ) ) ;
#11162=ORIENTED_EDGE ( 'NONE', *, *, #740, .F. ) ;
#11163=CARTESIAN_POINT ( 'NONE',  ( 65.26950693702184481, -11.12283941681556954, 72.18019809873047166 ) ) ;
#11168=FACE_OUTER_BOUND ( 'NONE', #4120, .T. ) ;
#11173=LINE ( 'NONE', #1855, #910 ) ;
#11177=CARTESIAN_POINT ( 'NONE',  ( 53.11142512232702018, -3.558169932106523881, 62.84860122826521689 ) ) ;
#11179=CARTESIAN_POINT ( 'NONE',  ( 55.09646579789918519, -6.394265699299607419, 62.84860122826521689 ) ) ;
#11180=ORIENTED_EDGE ( 'NONE', *, *, #9195, .F. ) ;
#11185=VERTEX_POINT ( 'NONE', #12780 ) ;
#11189=EDGE_CURVE ( 'NONE', #9615, #556, #10232, .T. ) ;
#11192=AXIS2_PLACEMENT_3D ( 'NONE', #10871, #14409, #4868 ) ;
#11197=ORIENTED_EDGE ( 'NONE', *, *, #15171, .F. ) ;
#11205=CARTESIAN_POINT ( 'NONE',  ( 69.46451213741848107, -2.308034861962666717, 72.93576380291801797 ) ) ;
#11215=CARTESIAN_POINT ( 'NONE',  ( 61.18622467607353599, 2.299242679852274929, 48.51982618741349285 ) ) ;
#11220=VERTEX_POINT ( 'NONE', #1140 ) ;
#11222=EDGE_CURVE ( 'NONE', #9708, #3099, #6013, .T. ) ;
#11225=VECTOR ( 'NONE', #10661, 1000.000000000000114 ) ;
#11226=DIRECTION ( 'NONE',  ( -0.01745240642731254316, 0.9998476951565652415, 0.000000000000000000 ) ) ;
#11227=CARTESIAN_POINT ( 'NONE',  ( 71.76344687472122530, -15.59526412071138957, 73.07464432123545350 ) ) ;
#11229=CARTESIAN_POINT ( 'NONE',  ( 62.80738265182633739, -4.914066317053380040, 87.40005259842790508 ) ) ;
#11231=AXIS2_PLACEMENT_3D ( 'NONE', #14974, #11500, #4422 ) ;
#11232=CARTESIAN_POINT ( 'NONE',  ( 65.81539560090801899, -11.71715063578952964, 72.32462332011485273 ) ) ;
#11233=CARTESIAN_POINT ( 'NONE',  ( 69.30413741146281836, -4.165477212746960589, 77.19766410831375936 ) ) ;
#11235=CARTESIAN_POINT ( 'NONE',  ( 66.38598137497019991, -11.47113225237460910, 76.19766410831374515 ) ) ;
#11245=AXIS2_PLACEMENT_3D ( 'NONE', #2081, #3395, #11699 ) ;
#11250=DIRECTION ( 'NONE',  ( 0.000000000000000000, 0.000000000000000000, 1.000000000000000000 ) ) ;
#11256=CARTESIAN_POINT ( 'NONE',  ( 58.00000000000000711, -2.249290599286309256, 87.40005259842790508 ) ) ;
#11262=CARTESIAN_POINT ( 'NONE',  ( 70.46453521882888538, -2.298370886119716960, 73.19766410831374515 ) ) ;
#11263=LINE ( 'NONE', #9906, #3641 ) ;
#11264=CARTESIAN_POINT ( 'NONE',  ( 58.00000000000000711, -2.249290599286309256, 81.40005259842790508 ) ) ;
#11267=ORIENTED_EDGE ( 'NONE', *, *, #9044, .T. ) ;
#11272=ORIENTED_EDGE ( 'NONE', *, *, #1068, .T. ) ;
#11274=CARTESIAN_POINT ( 'NONE',  ( 52.50499674461036648, -3.053107681157296582, 48.51982618741349285 ) ) ;
#11278=ADVANCED_FACE ( 'NONE', ( #12216 ), #5142, .T. ) ;
#11288=DIRECTION ( 'NONE',  ( 0.4848096202550660205, 0.8746197071345573892, 0.000000000000000000 ) ) ;
#11294=ORIENTED_EDGE ( 'NONE', *, *, #12710, .T. ) ;
#11297=AXIS2_PLACEMENT_3D ( 'NONE', #7459, #3684, #11837 ) ;
#11303=CARTESIAN_POINT ( 'NONE',  ( 70.25075942771931636, -4.321398257530866260, 76.19766410831374515 ) ) ;
#11304=CARTESIAN_POINT ( 'NONE',  ( 69.46454297106443221, -2.294433322023680333, 75.32995078675688205 ) ) ;
#11309=CARTESIAN_POINT ( 'NONE',  ( 69.97972560191894331, -3.172990595108510004, 73.12858342702070047 ) ) ;
#11313=CARTESIAN_POINT ( 'NONE',  ( 58.14816640453862107, 2.809303687574978614, 48.51982618741349285 ) ) ;
#11321=DIRECTION ( 'NONE',  ( 0.1334096321106371386, -0.9910609820087281641, 0.000000000000000000 ) ) ;
#11322=FACE_OUTER_BOUND ( 'NONE', #10134, .T. ) ;
#11325=ORIENTED_EDGE ( 'NONE', *, *, #9488, .T. ) ;
#11327=VERTEX_POINT ( 'NONE', #5217 ) ;
#11331=ORIENTED_EDGE ( 'NONE', *, *, #1119, .F. ) ;
#11334=DIRECTION ( 'NONE',  ( 0.000000000000000000, 0.000000000000000000, 1.000000000000000000 ) ) ;
#11336=CIRCLE ( 'NONE', #4724, 0.7892041907098306108 ) ;
#11339=EDGE_CURVE ( 'NONE', #3036, #3165, #8524, .T. ) ;
#11348=VECTOR ( 'NONE', #84, 1000.000000000000000 ) ;
#11350=VERTEX_POINT ( 'NONE', #7381 ) ;
#11354=DIRECTION ( 'NONE',  ( -1.000000000000000000, 0.000000000000000000, 0.000000000000000000 ) ) ;
#11370=ORIENTED_EDGE ( 'NONE', *, *, #12920, .T. ) ;
#11384=DIRECTION ( 'NONE',  ( 0.3020115420618285085, -0.1674077314120178406, 0.9384901064608609511 ) ) ;
#11392=( NAMED_UNIT ( * ) SI_UNIT ( $, .STERADIAN. ) SOLID_ANGLE_UNIT ( ) );
#11402=ORIENTED_EDGE ( 'NONE', *, *, #10547, .T. ) ;
#11412=DIRECTION ( 'NONE',  ( -0.000000000000000000, 0.000000000000000000, -1.000000000000000000 ) ) ;
#11421=CARTESIAN_POINT ( 'NONE',  ( 50.19487218104683990, 2.077162398607073079, 47.51982618741348574 ) ) ;
#11423=DIRECTION ( 'NONE',  ( 0.000000000000000000, 0.000000000000000000, 1.000000000000000000 ) ) ;
#11431=APPLICATION_CONTEXT ( 'automotive_design' ) ;
#11434=DIRECTION ( 'NONE',  ( 0.000000000000000000, 0.000000000000000000, 1.000000000000000000 ) ) ;
#11435=FACE_OUTER_BOUND ( 'NONE', #14036, .T. ) ;
#11436=EDGE_LOOP ( 'NONE', ( #2188, #7783 ) ) ;
#11438=ORIENTED_EDGE ( 'NONE', *, *, #4617, .T. ) ;
#11452=CARTESIAN_POINT ( 'NONE',  ( 62.14609464170151654, 0.6526447315840442354, 48.51982618741349285 ) ) ;
#11453=CARTESIAN_POINT ( 'NONE',  ( 64.61411691048888883, -11.63232581132101195, 73.01473414043169896 ) ) ;
#11458=ORIENTED_EDGE ( 'NONE', *, *, #13140, .T. ) ;
#11459=CARTESIAN_POINT ( 'NONE',  ( 69.28051765693513175, -4.295678830383772961, 71.19766410831373094 ) ) ;
#11468=DIRECTION ( 'NONE',  ( 0.9991708782893151675, -0.04071309345356645404, 0.000000000000000000 ) ) ;
#11472=DIRECTION ( 'NONE',  ( 0.000000000000000000, 0.000000000000000000, -1.000000000000000000 ) ) ;
#11473=EDGE_CURVE ( 'NONE', #13714, #931, #5444, .T. ) ;
#11474=ADVANCED_FACE ( 'NONE', ( #7984 ), #7833, .T. ) ;
#11485=DIRECTION ( 'NONE',  ( 0.8746197071345573892, -0.4848096202550657985, 0.000000000000000000 ) ) ;
#11500=DIRECTION ( 'NONE',  ( 0.000000000000000000, 0.000000000000000000, 1.000000000000000000 ) ) ;
#11506=DIRECTION ( 'NONE',  ( 0.7915791710638007128, 0.6110666215217015473, 0.000000000000000000 ) ) ;
#11507=CARTESIAN_POINT ( 'NONE',  ( 120.5019411979502451, -32.32126606797570645, 54.40673322733726991 ) ) ;
#11509=ORIENTED_EDGE ( 'NONE', *, *, #2453, .T. ) ;
#11516=EDGE_CURVE ( 'NONE', #15000, #211, #11716, .T. ) ;
#11521=CARTESIAN_POINT ( 'NONE',  ( 63.55116547662790794, -2.088839582009629936, 60.61639468829817190 ) ) ;
#11525=EDGE_CURVE ( 'NONE', #10265, #3380, #10244, .T. ) ;
#11528=LINE ( 'NONE', #985, #5204 ) ;
#11534=CARTESIAN_POINT ( 'NONE',  ( 69.46373470288038732, -2.401743389192480649, 75.84280485847520481 ) ) ;
#11535=DIRECTION ( 'NONE',  ( 0.000000000000000000, 0.000000000000000000, 1.000000000000000000 ) ) ;
#11544=VERTEX_POINT ( 'NONE', #1824 ) ;
#11552=CARTESIAN_POINT ( 'NONE',  ( 70.26445833701072274, -4.474174595298148205, 77.19766410831374515 ) ) ;
#11553=DIRECTION ( 'NONE',  ( -0.8746197071345569451, 0.4848096202550666312, 0.000000000000000000 ) ) ;
#11559=AXIS2_PLACEMENT_3D ( 'NONE', #1901, #13310, #6380 ) ;
#11566=ADVANCED_FACE ( 'NONE', ( #7907 ), #6591, .T. ) ;
#11567=ADVANCED_FACE ( 'NONE', ( #6743 ), #2035, .F. ) ;
#11568=ORIENTED_EDGE ( 'NONE', *, *, #2311, .F. ) ;
#11569=FACE_OUTER_BOUND ( 'NONE', #7777, .T. ) ;
#11572=FACE_OUTER_BOUND ( 'NONE', #8229, .T. ) ;
#11574=CIRCLE ( 'NONE', #8398, 0.7892041907098262810 ) ;
#11588=VERTEX_POINT ( 'NONE', #9742 ) ;
#11591=DIRECTION ( 'NONE',  ( 1.000000000000000000, 0.000000000000000000, 0.000000000000000000 ) ) ;
#11592=CARTESIAN_POINT ( 'NONE',  ( 58.00000000000000711, -2.249290599286309256, 87.40005259842790508 ) ) ;
#11596=AXIS2_PLACEMENT_3D ( 'NONE', #7387, #14947, #13868 ) ;
#11600=CARTESIAN_POINT ( 'NONE',  ( 76.14589960879430919, -7.734310727912411920, 76.19766410831374515 ) ) ;
#11602=ORIENTED_EDGE ( 'NONE', *, *, #2263, .F. ) ;
#11603=LINE ( 'NONE', #6233, #12967 ) ;
#11608=CIRCLE ( 'NONE', #3251, 0.7892041907098262810 ) ;
#11609=VERTEX_POINT ( 'NONE', #6124 ) ;
#11610=AXIS2_PLACEMENT_3D ( 'NONE', #1322, #14258, #3705 ) ;
#11613=ORIENTED_EDGE ( 'NONE', *, *, #4092, .T. ) ;
#11620=CARTESIAN_POINT ( 'NONE',  ( 65.13162939602317181, -11.91918766459985513, 73.19766410831374515 ) ) ;
#11624=CIRCLE ( 'NONE', #4999, 0.7892041907098262810 ) ;
#11626=AXIS2_PLACEMENT_3D ( 'NONE', #13019, #6250, #9477 ) ;
#11632=( NAMED_UNIT ( * ) SI_UNIT ( $, .STERADIAN. ) SOLID_ANGLE_UNIT ( ) );
#11638=CIRCLE ( 'NONE', #11884, 0.7892041907098261699 ) ;
#11642=CYLINDRICAL_SURFACE ( 'NONE', #10056, 0.7892041907098262810 ) ;
#11644=DIRECTION ( 'NONE',  ( -0.8746197071345569451, 0.4848096202550666312, 0.000000000000000000 ) ) ;
#11645=ORIENTED_EDGE ( 'NONE', *, *, #8411, .T. ) ;
#11646=DIRECTION ( 'NONE',  ( -0.3020115420618265656, 0.1674077314120193949, -0.9384901064608611732 ) ) ;
#11660=EDGE_CURVE ( 'NONE', #3099, #931, #3613, .T. ) ;
#11676=EDGE_CURVE ( 'NONE', #3217, #10912, #10224, .T. ) ;
#11677=EDGE_CURVE ( 'NONE', #5032, #3522, #12490, .T. ) ;
#11686=VERTEX_POINT ( 'NONE', #483 ) ;
#11689=LINE ( 'NONE', #8322, #13820 ) ;
#11691=DIRECTION ( 'NONE',  ( -0.000000000000000000, 0.000000000000000000, -1.000000000000000000 ) ) ;
#11695=CARTESIAN_POINT ( 'NONE',  ( 65.17358638046424346, -11.90957281131293932, 72.92467134341568169 ) ) ;
#11699=DIRECTION ( 'NONE',  ( 0.8746197071345563900, -0.4848096202550675193, 0.000000000000000000 ) ) ;
#11702=ORIENTED_EDGE ( 'NONE', *, *, #5178, .T. ) ;
#11704=DIRECTION ( 'NONE',  ( -0.8208219420614780715, 0.4549890321264283277, 0.3453061251629916950 ) ) ;
#11716=CIRCLE ( 'NONE', #412, 1.000000000000002665 ) ;
#11731=AXIS2_PLACEMENT_3D ( 'NONE', #697, #2860, #8568 ) ;
#11732=DIRECTION ( 'NONE',  ( 0.4848096202550659650, 0.8746197071345572782, 0.000000000000000000 ) ) ;
#11735=CARTESIAN_POINT ( 'NONE',  ( 55.36337191871069763, -7.136966431295542534, 54.56811043785582882 ) ) ;
#11737=ADVANCED_FACE ( 'NONE', ( #11101 ), #14498, .F. ) ;
#11748=DIRECTION ( 'NONE',  ( 0.8746197071345582774, -0.4848096202550639666, 0.000000000000000000 ) ) ;
#11750=VECTOR ( 'NONE', #6620, 1000.000000000000000 ) ;
#11759=ORIENTED_EDGE ( 'NONE', *, *, #14969, .T. ) ;
#11761=ORIENTED_EDGE ( 'NONE', *, *, #364, .F. ) ;
#11764=EDGE_LOOP ( 'NONE', ( #12761, #2085, #10967, #8796 ) ) ;
#11769=LINE ( 'NONE', #5932, #11348 ) ;
#11780=CARTESIAN_POINT ( 'NONE',  ( 58.80593636315131079, 3.245402227105440129, 54.56811043785582882 ) ) ;
#11781=CIRCLE ( 'NONE', #13261, 0.9999999999999957812 ) ;
#11785=FACE_OUTER_BOUND ( 'NONE', #10340, .T. ) ;
#11786=DIRECTION ( 'NONE',  ( -0.8746197071345569451, 0.4848096202550666312, 0.000000000000000000 ) ) ;
#11791=DIRECTION ( 'NONE',  ( -0.000000000000000000, 0.000000000000000000, -1.000000000000000000 ) ) ;
#11794=AXIS2_PLACEMENT_3D ( 'NONE', #10591, #13055, #5909 ) ;
#11801=LINE ( 'NONE', #4806, #7301 ) ;
#11803=CIRCLE ( 'NONE', #11297, 12.46463184759104870 ) ;
#11804=CARTESIAN_POINT ( 'NONE',  ( 69.46156643657255358, -2.520042852607651263, 76.11175476292719111 ) ) ;
#11816=ORIENTED_EDGE ( 'NONE', *, *, #1419, .T. ) ;
#11821=ADVANCED_FACE ( 'NONE', ( #10486 ), #6784, .T. ) ;
#11822=AXIS2_PLACEMENT_3D ( 'NONE', #3729, #11891, #3803 ) ;
#11827=AXIS2_PLACEMENT_3D ( 'NONE', #11256, #7731, #11485 ) ;
#11832=CARTESIAN_POINT ( 'NONE',  ( 64.68829635872748440, -11.56127715054218008, 76.69739539199261458 ) ) ;
#11836=ORIENTED_EDGE ( 'NONE', *, *, #7726, .F. ) ;
#11837=DIRECTION ( 'NONE',  ( -0.8746197071345572782, 0.4848096202550660205, 0.000000000000000000 ) ) ;
#11840=AXIS2_PLACEMENT_3D ( 'NONE', #3397, #10635, #6939 ) ;
#11842=CARTESIAN_POINT ( 'NONE',  ( 56.28732689558331259, 3.089731932287651084, 60.61639468829817190 ) ) ;
#11851=CARTESIAN_POINT ( 'NONE',  ( 52.42117158417902800, -3.175556148104785148, 48.51982618741349285 ) ) ;
#11853=ORIENTED_EDGE ( 'NONE', *, *, #9692, .F. ) ;
#11858=ORIENTED_EDGE ( 'NONE', *, *, #5283, .T. ) ;
#11867=AXIS2_PLACEMENT_3D ( 'NONE', #795, #15044, #14879 ) ;
#11875=CARTESIAN_POINT ( 'NONE',  ( 54.07385127050791596, 1.678372679529495981, 48.51982618741349285 ) ) ;
#11879=APPLICATION_CONTEXT ( 'automotive_design' ) ;
#11880=ORIENTED_EDGE ( 'NONE', *, *, #8882, .T. ) ;
#11884=AXIS2_PLACEMENT_3D ( 'NONE', #13290, #367, #2527 ) ;
#11891=DIRECTION ( 'NONE',  ( 0.000000000000000000, 0.000000000000000000, -1.000000000000000000 ) ) ;
#11897=CARTESIAN_POINT ( 'NONE',  ( 65.80512781895316721, -6.575743597179694255, 47.51982618741348574 ) ) ;
#11899=CARTESIAN_POINT ( 'NONE',  ( 64.71404714396263103, -11.54274494033589704, 76.72447063483126328 ) ) ;
#11904=LINE ( 'NONE', #6067, #1664 ) ;
#11909=EDGE_CURVE ( 'NONE', #10912, #6596, #7872, .T. ) ;
#11916=DIRECTION ( 'NONE',  ( -0.8746197071345569451, 0.4848096202550666312, 0.000000000000000000 ) ) ;
#11917=VERTEX_POINT ( 'NONE', #6710 ) ;
#11922=DIRECTION ( 'NONE',  ( -0.6727821148276317276, 0.7398406760702329610, 0.000000000000000000 ) ) ;
#11926=CARTESIAN_POINT ( 'NONE',  ( 66.11195137528358146, -11.60156588980731485, 72.22102352638243872 ) ) ;
#11945=AXIS2_PLACEMENT_3D ( 'NONE', #14332, #889, #11506 ) ;
#11953=ADVANCED_FACE ( 'NONE', ( #9728 ), #10795, .T. ) ;
#11954=CARTESIAN_POINT ( 'NONE',  ( 69.99380555487256572, -3.213667230009126463, 75.47065687321054384 ) ) ;
#11957=CIRCLE ( 'NONE', #3847, 4.496540510819673209 ) ;
#11969=CARTESIAN_POINT ( 'NONE',  ( 66.38598137497019991, -11.47113225237460377, 76.19766410831375936 ) ) ;
#11970=EDGE_LOOP ( 'NONE', ( #4308, #14016, #11370, #11458 ) ) ;
#11971=DIRECTION ( 'NONE',  ( 1.000000000000000000, 0.000000000000000000, 0.000000000000000000 ) ) ;
#11972=SHAPE_REPRESENTATION ( 'Locking Handle', ( #6315 ), #4840 ) ;
#11975=AXIS2_PLACEMENT_3D ( 'NONE', #15202, #6806, #15050 ) ;
#11977=CIRCLE ( 'NONE', #2652, 0.7892041907098256148 ) ;
#11982=CARTESIAN_POINT ( 'NONE',  ( 52.72354942432796321, 0.2729788054883388049, 48.51982618741349285 ) ) ;
#11984=CYLINDRICAL_SURFACE ( 'NONE', #999, 0.7892041907098262810 ) ;
#11989=AXIS2_PLACEMENT_3D ( 'NONE', #11552, #2176, #860 ) ;
#11998=CIRCLE ( 'NONE', #12244, 0.7892041907098303888 ) ;
#12006=CARTESIAN_POINT ( 'NONE',  ( 34.14268298385128730, 5.258265827056129993, 91.03215601016300695 ) ) ;
#12007=CARTESIAN_POINT ( 'NONE',  ( 72.56943418881560603, -14.89867611640088896, 76.13615421477460643 ) ) ;
#12011=CARTESIAN_POINT ( 'NONE',  ( 57.26556849154462725, -7.256479411572841265, 62.84860122826521689 ) ) ;
#12018=DIRECTION ( 'NONE',  ( 0.8746197071345560570, -0.4848096202550682410, 0.000000000000000000 ) ) ;
#12022=CIRCLE ( 'NONE', #14719, 0.7892041907098273912 ) ;
#12023=LINE ( 'NONE', #1408, #14008 ) ;
#12027=DIRECTION ( 'NONE',  ( 0.8208219420614810691, -0.4549890321264228876, -0.3453061251629915285 ) ) ;
#12028=LINE ( 'NONE', #14124, #7306 ) ;
#12029=CARTESIAN_POINT ( 'NONE',  ( 69.36169026123523906, -3.800370218431805114, 77.14753538332058724 ) ) ;
#12035=CARTESIAN_POINT ( 'NONE',  ( 64.79680489028815771, -11.48253646253152560, 71.59064503457959461 ) ) ;
#12038=CARTESIAN_POINT ( 'NONE',  ( 57.51704887355756313, 3.283153786997079049, 48.51982618741349285 ) ) ;
#12043=ORIENTED_EDGE ( 'NONE', *, *, #10223, .F. ) ;
#12045=CIRCLE ( 'NONE', #7139, 4.999999999999997335 ) ;
#12046=ORIENTED_EDGE ( 'NONE', *, *, #2458, .T. ) ;
#12050=DIRECTION ( 'NONE',  ( -0.8746197071345571672, 0.4848096202550659650, 0.000000000000000000 ) ) ;
#12060=ORIENTED_EDGE ( 'NONE', *, *, #6369, .F. ) ;
#12062=EDGE_CURVE ( 'NONE', #3816, #10484, #10085, .T. ) ;
#12063=CARTESIAN_POINT ( 'NONE',  ( 58.00000000000000711, -2.249290599286309256, 47.51982618741348574 ) ) ;
#12064=ORIENTED_EDGE ( 'NONE', *, *, #1792, .T. ) ;
#12068=ORIENTED_EDGE ( 'NONE', *, *, #2886, .T. ) ;
#12078=ORIENTED_EDGE ( 'NONE', *, *, #5025, .F. ) ;
#12081=CARTESIAN_POINT ( 'NONE',  ( 58.00000000000000711, -2.249290599286309256, 82.40005259842790508 ) ) ;
#12088=EDGE_CURVE ( 'NONE', #153, #7206, #6764, .T. ) ;
#12089=ORIENTED_EDGE ( 'NONE', *, *, #8499, .T. ) ;
#12090=AXIS2_PLACEMENT_3D ( 'NONE', #635, #7732, #2878 ) ;
#12096=DIRECTION ( 'NONE',  ( 0.8746197071345571672, -0.4848096202550661316, 0.000000000000000000 ) ) ;
#12099=VERTEX_POINT ( 'NONE', #6534 ) ;
#12102=DIRECTION ( 'NONE',  ( -0.000000000000000000, 0.000000000000000000, -1.000000000000000000 ) ) ;
#12106=VECTOR ( 'NONE', #12166, 1000.000000000000000 ) ;
#12111=DIRECTION ( 'NONE',  ( -0.000000000000000000, 0.000000000000000000, -1.000000000000000000 ) ) ;
#12115=CARTESIAN_POINT ( 'NONE',  ( 69.43180921594577626, -3.262091255642812992, 75.98418538769692532 ) ) ;
#12128=VERTEX_POINT ( 'NONE', #2785 ) ;
#12132=DIRECTION ( 'NONE',  ( -0.8746197071345572782, 0.4848096202550659650, 0.000000000000000000 ) ) ;
#12133=ORIENTED_EDGE ( 'NONE', *, *, #11025, .T. ) ;
#12135=VECTOR ( 'NONE', #517, 1000.000000000000000 ) ;
#12139=ADVANCED_FACE ( 'NONE', ( #6392 ), #7765, .F. ) ;
#12140=VERTEX_POINT ( 'NONE', #7481 ) ;
#12141=VERTEX_POINT ( 'NONE', #682 ) ;
#12146=ORIENTED_EDGE ( 'NONE', *, *, #6687, .T. ) ;
#12148=ORIENTED_EDGE ( 'NONE', *, *, #5371, .F. ) ;
#12151=ORIENTED_EDGE ( 'NONE', *, *, #11473, .F. ) ;
#12160=CARTESIAN_POINT ( 'NONE',  ( 61.57781019154727176, -5.828480965243416634, 60.61639468829817190 ) ) ;
#12166=DIRECTION ( 'NONE',  ( 0.000000000000000000, 0.000000000000000000, 1.000000000000000000 ) ) ;
#12190=CARTESIAN_POINT ( 'NONE',  ( 58.00000000000000711, -2.249290599286309256, 38.50000000000012790 ) ) ;
#12196=CARTESIAN_POINT ( 'NONE',  ( 71.80003071982790175, -14.47218880931180962, 73.19766410831374515 ) ) ;
#12200=AXIS2_PLACEMENT_3D ( 'NONE', #1191, #4886, #12972 ) ;
#12203=AXIS2_PLACEMENT_3D ( 'NONE', #3942, #5409, #5179 ) ;
#12206=CIRCLE ( 'NONE', #10245, 11.46463184759104870 ) ;
#12214=VERTEX_POINT ( 'NONE', #12625 ) ;
#12216=FACE_OUTER_BOUND ( 'NONE', #13511, .T. ) ;
#12232=TOROIDAL_SURFACE ( 'NONE', #5604, 10.46463184759104870, 1.000000000000000000 ) ;
#12235=CIRCLE ( 'NONE', #5606, 0.9999999999999954481 ) ;
#12236=EDGE_CURVE ( 'NONE', #9304, #12214, #11528, .T. ) ;
#12238=ORIENTED_EDGE ( 'NONE', *, *, #2256, .T. ) ;
#12244=AXIS2_PLACEMENT_3D ( 'NONE', #13478, #12554, #4304 ) ;
#12254=ORIENTED_EDGE ( 'NONE', *, *, #6154, .T. ) ;
#12256=FACE_OUTER_BOUND ( 'NONE', #8459, .T. ) ;
#12257=ORIENTED_EDGE ( 'NONE', *, *, #5611, .T. ) ;
#12258=EDGE_CURVE ( 'NONE', #11609, #9619, #1073, .T. ) ;
#12262=DIRECTION ( 'NONE',  ( 0.000000000000000000, 0.000000000000000000, 1.000000000000000000 ) ) ;
#12263=AXIS2_PLACEMENT_3D ( 'NONE', #6846, #3159, #10014 ) ;
#12268=CARTESIAN_POINT ( 'NONE',  ( 62.14930354033766946, 1.441842398587370067, 60.61639468829817190 ) ) ;
#12270=VERTEX_POINT ( 'NONE', #9082 ) ;
#12282=VERTEX_POINT ( 'NONE', #14088 ) ;
#12293=CARTESIAN_POINT ( 'NONE',  ( 54.21883389619742388, -5.612936290787406968, 60.61639468829817190 ) ) ;
#12301=CARTESIAN_POINT ( 'NONE',  ( 53.11142512232702018, -3.558169932106523881, 60.61639468829817190 ) ) ;
#12313=CYLINDRICAL_SURFACE ( 'NONE', #10632, 0.7892041907098262810 ) ;
#12314=CARTESIAN_POINT ( 'NONE',  ( 60.65595175199513278, -6.557103238384438981, 48.51982618741349285 ) ) ;
#12319=CARTESIAN_POINT ( 'NONE',  ( 65.88530916257730041, -11.69141299361105979, 72.29513642469299839 ) ) ;
#12320=DIRECTION ( 'NONE',  ( -0.9876883405935777960, 0.1564344650500800460, 0.000000000000000000 ) ) ;
#12321=DIRECTION ( 'NONE',  ( -0.000000000000000000, 0.000000000000000000, -1.000000000000000000 ) ) ;
#12324=AXIS2_PLACEMENT_3D ( 'NONE', #4586, #3520, #8221 ) ;
#12333=ORIENTED_EDGE ( 'NONE', *, *, #7345, .F. ) ;
#12335=( GEOMETRIC_REPRESENTATION_CONTEXT ( 3 ) GLOBAL_UNCERTAINTY_ASSIGNED_CONTEXT ( ( #14435 ) ) GLOBAL_UNIT_ASSIGNED_CONTEXT ( ( #2945, #6546, #11392 ) ) REPRESENTATION_CONTEXT ( 'NONE', 'WORKASPACE' ) );
#12336=AXIS2_PLACEMENT_3D ( 'NONE', #4804, #8276, #4957 ) ;
#12350=ORIENTED_EDGE ( 'NONE', *, *, #4537, .T. ) ;
#12357=DIRECTION ( 'NONE',  ( -0.000000000000000000, 0.000000000000000000, -1.000000000000000000 ) ) ;
#12360=EDGE_CURVE ( 'NONE', #3217, #8760, #3691, .T. ) ;
#12365=EDGE_CURVE ( 'NONE', #1600, #5032, #7661, .T. ) ;
#12367=CARTESIAN_POINT ( 'NONE',  ( 120.4255624041552721, -41.42576115427227990, 51.74171249506144932 ) ) ;
#12368=ORIENTED_EDGE ( 'NONE', *, *, #6154, .F. ) ;
#12376=ORIENTED_EDGE ( 'NONE', *, *, #9720, .T. ) ;
#12392=EDGE_LOOP ( 'NONE', ( #3393, #281, #650, #4291, #7591 ) ) ;
#12393=EDGE_CURVE ( 'NONE', #3816, #12099, #1016, .T. ) ;
#12395=CARTESIAN_POINT ( 'NONE',  ( 65.71319926014257362, -10.73129157630437724, 71.19766410831374515 ) ) ;
#12397=FACE_OUTER_BOUND ( 'NONE', #4150, .T. ) ;
#12404=CARTESIAN_POINT ( 'NONE',  ( 47.97280705105441001, 3.308873213108443512, 82.40005259842790508 ) ) ;
#12409=DIRECTION ( 'NONE',  ( 0.000000000000000000, 0.000000000000000000, 1.000000000000000000 ) ) ;
#12410=PLANE ( 'NONE',  #6858 ) ;
#12411=DIRECTION ( 'NONE',  ( -0.8746197071345569451, 0.4848096202550666312, 0.000000000000000000 ) ) ;
#12417=CARTESIAN_POINT ( 'NONE',  ( 59.59091026602544616, -7.053490217115945704, 62.84860122826521689 ) ) ;
#12435=LINE ( 'NONE', #1889, #5920 ) ;
#12438=DIRECTION ( 'NONE',  ( -0.3020115420618161295, 0.1674077314120152038, -0.9384901064608655030 ) ) ;
#12440=ORIENTED_EDGE ( 'NONE', *, *, #13013, .F. ) ;
#12449=DIRECTION ( 'NONE',  ( 0.000000000000000000, 0.000000000000000000, 1.000000000000000000 ) ) ;
#12454=FACE_OUTER_BOUND ( 'NONE', #3336, .T. ) ;
#12459=AXIS2_PLACEMENT_3D ( 'NONE', #9590, #2578, #8356 ) ;
#12469=CARTESIAN_POINT ( 'NONE',  ( 64.36032056549935021, -11.78815919431190196, 72.16553326196626017 ) ) ;
#12490=LINE ( 'NONE', #8638, #7030 ) ;
#12492=DIRECTION ( 'NONE',  ( 0.000000000000000000, 0.000000000000000000, 1.000000000000000000 ) ) ;
#12498=DIRECTION ( 'NONE',  ( 0.8746197071345590546, -0.4848096202550629674, 0.000000000000000000 ) ) ;
#12501=DIRECTION ( 'NONE',  ( -1.000000000000000000, 0.000000000000000000, 0.000000000000000000 ) ) ;
#12511=ORIENTED_EDGE ( 'NONE', *, *, #10450, .T. ) ;
#12515=ADVANCED_FACE ( 'NONE', ( #819 ), #7911, .T. ) ;
#12517=CIRCLE ( 'NONE', #8818, 0.7892041907098322762 ) ;
#12522=DIRECTION ( 'NONE',  ( -0.000000000000000000, 0.000000000000000000, -1.000000000000000000 ) ) ;
#12528=VECTOR ( 'NONE', #11646, 1000.000000000000114 ) ;
#12529=EDGE_CURVE ( 'NONE', #10265, #7295, #13069, .T. ) ;
#12541=DIRECTION ( 'NONE',  ( 0.000000000000000000, 0.000000000000000000, 1.000000000000000000 ) ) ;
#12547=ORIENTED_EDGE ( 'NONE', *, *, #7999, .T. ) ;
#12554=DIRECTION ( 'NONE',  ( 0.000000000000000000, 0.000000000000000000, 1.000000000000000000 ) ) ;
#12560=TOROIDAL_SURFACE ( 'NONE', #5939, 12.46463184759105047, 1.000000000000000000 ) ;
#12564=CARTESIAN_POINT ( 'NONE',  ( 76.63070922904938698, -6.859691020777852977, 76.19766410831374515 ) ) ;
#12569=FACE_OUTER_BOUND ( 'NONE', #3367, .T. ) ;
#12570=AXIS2_PLACEMENT_3D ( 'NONE', #9192, #6870, #5738 ) ;
#12572=CIRCLE ( 'NONE', #5954, 1.000000000000000888 ) ;
#12575=LINE ( 'NONE', #9266, #12528 ) ;
#12576=ORIENTED_EDGE ( 'NONE', *, *, #11660, .T. ) ;
#12577=CARTESIAN_POINT ( 'NONE',  ( 75.67850768186842458, -7.475231152235347842, 72.19766410831374515 ) ) ;
#12579=EDGE_LOOP ( 'NONE', ( #10308, #13879, #6254, #3588 ) ) ;
#12580=STYLED_ITEM('',(#15279),#14200);
#12581=CARTESIAN_POINT ( 'NONE',  ( 120.1999296558884254, -32.15385833656369385, 53.46824312087640863 ) ) ;
#12583=AXIS2_PLACEMENT_3D ( 'NONE', #12417, #1867, #5344 ) ;
#12584=AXIS2_PLACEMENT_3D ( 'NONE', #3342, #8043, #1033 ) ;
#12586=CARTESIAN_POINT ( 'NONE',  ( 58.00000000000000711, -2.249290599286309256, 47.51982618741348574 ) ) ;
#12588=CARTESIAN_POINT ( 'NONE',  ( 68.96257531573284894, -3.752529052654163255, 76.19766410831374515 ) ) ;
#12589=DIRECTION ( 'NONE',  ( 0.8746197071345570562, -0.4848096202550665756, 0.000000000000000000 ) ) ;
#12590=VECTOR ( 'NONE', #11041, 1000.000000000000000 ) ;
#12592=CIRCLE ( 'NONE', #9162, 0.7892041907098322762 ) ;
#12594=AXIS2_PLACEMENT_3D ( 'NONE', #2089, #10181, #9016 ) ;
#12600=CARTESIAN_POINT ( 'NONE',  ( 66.38598137497019991, -11.47113225237460910, 77.19766410831374515 ) ) ;
#12601=CARTESIAN_POINT ( 'NONE',  ( 58.00000000000000711, -2.249290599286309256, 81.40005259842790508 ) ) ;
#12603=CARTESIAN_POINT ( 'NONE',  ( 55.86211336638498182, 2.337731330496643167, 62.84860122826521689 ) ) ;
#12611=CARTESIAN_POINT ( 'NONE',  ( 52.83848824477699679, -4.298675648159541396, 60.61639468829817190 ) ) ;
#12618=ORIENTED_EDGE ( 'NONE', *, *, #9899, .F. ) ;
#12619=AXIS2_PLACEMENT_3D ( 'NONE', #141, #5773, #15145 ) ;
#12625=CARTESIAN_POINT ( 'NONE',  ( 54.00000000000000711, -2.249290599286310588, 38.50000000000012790 ) ) ;
#12629=DIRECTION ( 'NONE',  ( 0.8746197071345569451, -0.4848096202550666312, 0.000000000000000000 ) ) ;
#12630=CARTESIAN_POINT ( 'NONE',  ( 69.46451111827113323, -2.308386634095125345, 75.46236687596045556 ) ) ;
#12644=ADVANCED_FACE ( 'NONE', ( #14646 ), #3490, .T. ) ;
#12647=DIRECTION ( 'NONE',  ( 0.8746197071345590546, -0.4848096202550629674, 0.000000000000000000 ) ) ;
#12648=CARTESIAN_POINT ( 'NONE',  ( 53.11142512232702018, -3.558169932106523881, 48.51982618741349285 ) ) ;
#12656=CARTESIAN_POINT ( 'NONE',  ( 52.94134894379979528, -2.395505968190773327, 62.84860122826521689 ) ) ;
#12658=DIRECTION ( 'NONE',  ( 0.000000000000000000, 0.000000000000000000, 1.000000000000000000 ) ) ;
#12660=ADVANCED_FACE ( 'NONE', ( #8582 ), #13415, .T. ) ;
#12664=DIRECTION ( 'NONE',  ( -0.8746197071345572782, 0.4848096202550659650, -0.000000000000000000 ) ) ;
#12680=CARTESIAN_POINT ( 'NONE',  ( 58.00000000000000711, -2.249290599286309256, 87.40005259842790508 ) ) ;
#12684=DIRECTION ( 'NONE',  ( -0.8208219420614785156, 0.4549890321264268844, 0.3453061251629924167 ) ) ;
#12695=AXIS2_PLACEMENT_3D ( 'NONE', #756, #8995, #11226 ) ;
#12702=CARTESIAN_POINT ( 'NONE',  ( 56.97758043373130477, 2.707118148285912795, 60.61639468829817190 ) ) ;
#12706=CARTESIAN_POINT ( 'NONE',  ( 67.15257324181105503, -7.322644791425997113, 60.61639468829817190 ) ) ;
#12709=ORIENTED_EDGE ( 'NONE', *, *, #364, .T. ) ;
#12710=EDGE_CURVE ( 'NONE', #7295, #10265, #12846, .T. ) ;
#12711=CARTESIAN_POINT ( 'NONE',  ( 70.13908301581606963, -3.720822497039482979, 72.39370326752943186 ) ) ;
#12726=AXIS2_PLACEMENT_3D ( 'NONE', #7479, #11157, #14692 ) ;
#12727=DIRECTION ( 'NONE',  ( 0.000000000000000000, 0.000000000000000000, -1.000000000000000000 ) ) ;
#12730=CYLINDRICAL_SURFACE ( 'NONE', #13540, 0.7892041907098262810 ) ;
#12732=ORIENTED_EDGE ( 'NONE', *, *, #10509, .T. ) ;
#12747=DIRECTION ( 'NONE',  ( 0.8746197071345590546, -0.4848096202550629674, 0.000000000000000000 ) ) ;
#12759=ORIENTED_EDGE ( 'NONE', *, *, #2311, .T. ) ;
#12761=ORIENTED_EDGE ( 'NONE', *, *, #10646, .F. ) ;
#12777=DIRECTION ( 'NONE',  ( -0.000000000000000000, 0.000000000000000000, -1.000000000000000000 ) ) ;
#12780=CARTESIAN_POINT ( 'NONE',  ( 53.19261734817368392, 0.4154851184807644149, 82.40005259842790508 ) ) ;
#12789=DIRECTION ( 'NONE',  ( 0.3583679495359998191, -0.9335804265007718872, 0.000000000000000000 ) ) ;
#12807=EDGE_CURVE ( 'NONE', #7606, #14840, #12592, .T. ) ;
#12809=DIRECTION ( 'NONE',  ( 0.000000000000000000, 0.000000000000000000, 1.000000000000000000 ) ) ;
#12815=DIRECTION ( 'NONE',  ( 0.9839406800755992055, -0.1784957649143736891, 0.000000000000000000 ) ) ;
#12818=DIRECTION ( 'NONE',  ( -0.000000000000000000, 0.000000000000000000, -1.000000000000000000 ) ) ;
#12826=FACE_OUTER_BOUND ( 'NONE', #14580, .T. ) ;
#12836=AXIS2_PLACEMENT_3D ( 'NONE', #2230, #7566, #8999 ) ;
#12838=CARTESIAN_POINT ( 'NONE',  ( 70.46453521882889959, -2.298370886119723622, 82.40005259842790508 ) ) ;
#12840=CARTESIAN_POINT ( 'NONE',  ( 64.48276670783141640, -11.70694761207440671, 76.45535061892491058 ) ) ;
#12842=DIRECTION ( 'NONE',  ( 0.8208219420614785156, -0.4549890321264269399, -0.3453061251629920836 ) ) ;
#12846=CIRCLE ( 'NONE', #3981, 7.924024642120691908 ) ;
#12848=CIRCLE ( 'NONE', #6216, 0.7892041907098290565 ) ;
#12863=FACE_OUTER_BOUND ( 'NONE', #11040, .T. ) ;
#12866=CARTESIAN_POINT ( 'NONE',  ( 62.30678795759143185, -4.906903613034745426, 60.61639468829817190 ) ) ;
#12867=CARTESIAN_POINT ( 'NONE',  ( 70.17731411157174648, -3.883646954095939741, 72.30896232854578898 ) ) ;
#12869=ORIENTED_EDGE ( 'NONE', *, *, #8747, .T. ) ;
#12872=DIRECTION ( 'NONE',  ( 0.8746197071345569451, -0.4848096202550666312, 0.000000000000000000 ) ) ;
#12876=CIRCLE ( 'NONE', #13347, 1.000000000000007550 ) ;
#12880=FACE_OUTER_BOUND ( 'NONE', #6718, .T. ) ;
#12894=FACE_OUTER_BOUND ( 'NONE', #8986, .T. ) ;
#12910=ORIENTED_EDGE ( 'NONE', *, *, #4862, .F. ) ;
#12913=CARTESIAN_POINT ( 'NONE',  ( 71.15942379059755751, -15.26044865788734484, 72.19766410831374515 ) ) ;
#12918=CARTESIAN_POINT ( 'NONE',  ( 65.08836494111386628, -11.27206642318173735, 76.12732364699549237 ) ) ;
#12920=EDGE_CURVE ( 'NONE', #13229, #5503, #8427, .T. ) ;
#12930=FACE_OUTER_BOUND ( 'NONE', #13498, .T. ) ;
#12932=ADVANCED_FACE ( 'NONE', ( #8354 ), #4731, .T. ) ;
#12933=ORIENTED_EDGE ( 'NONE', *, *, #13360, .T. ) ;
#12934=CARTESIAN_POINT ( 'NONE',  ( 52.35373241494735197, -0.8423457118892130335, 62.84860122826521689 ) ) ;
#12939=VERTEX_POINT ( 'NONE', #9504 ) ;
#12946=CARTESIAN_POINT ( 'NONE',  ( 69.36166834748301824, -3.800326805936743213, 71.24799951533148601 ) ) ;
#12948=ORIENTED_EDGE ( 'NONE', *, *, #7672, .T. ) ;
#12949=EDGE_CURVE ( 'NONE', #59, #4156, #9893, .T. ) ;
#12951=DIRECTION ( 'NONE',  ( -0.000000000000000000, 0.000000000000000000, -1.000000000000000000 ) ) ;
#12960=AXIS2_PLACEMENT_3D ( 'NONE', #4199, #13521, #11354 ) ;
#12967=VECTOR ( 'NONE', #10919, 1000.000000000000000 ) ;
#12972=DIRECTION ( 'NONE',  ( 4.163336342344333240E-14, -2.515349040166368078E-14, 1.000000000000000000 ) ) ;
#12975=AXIS2_PLACEMENT_3D ( 'NONE', #1639, #1711, #7719 ) ;
#12976=CARTESIAN_POINT ( 'NONE',  ( 69.43927565506325550, -3.017240787745353980, 76.72358418092962040 ) ) ;
#12977=CARTESIAN_POINT ( 'NONE',  ( 75.52271037289314393, -7.388871293676331220, 71.19766410831374515 ) ) ;
#12986=LINE ( 'NONE', #12913, #13424 ) ;
#12993=DIRECTION ( 'NONE',  ( 0.8746197071345573892, -0.4848096202550657430, 0.000000000000000000 ) ) ;
#12994=AXIS2_PLACEMENT_3D ( 'NONE', #12160, #8332, #2554 ) ;
#12999=DIRECTION ( 'NONE',  ( 0.9111637130653279515, 0.4120445218577777902, 0.000000000000000000 ) ) ;
#13008=FACE_OUTER_BOUND ( 'NONE', #9770, .T. ) ;
#13011=DIRECTION ( 'NONE',  ( -0.000000000000000000, 0.000000000000000000, -1.000000000000000000 ) ) ;
#13013=EDGE_CURVE ( 'NONE', #5320, #14082, #6119, .T. ) ;
#13015=DIRECTION ( 'NONE',  ( 0.8746197071345570562, -0.4848096202550662981, 0.000000000000000000 ) ) ;
#13016=LINE ( 'NONE', #7004, #13086 ) ;
#13019=CARTESIAN_POINT ( 'NONE',  ( 65.92402464212069901, -2.249290599286309256, 39.50000000000012790 ) ) ;
#13021=CARTESIAN_POINT ( 'NONE',  ( 65.35437866493117554, -11.86302964528753634, 72.64181548138913058 ) ) ;
#13022=ORIENTED_EDGE ( 'NONE', *, *, #11222, .T. ) ;
#13023=CARTESIAN_POINT ( 'NONE',  ( 54.07385127050791596, 1.678372679529495981, 54.56811043785582882 ) ) ;
#13034=DIRECTION ( 'NONE',  ( -0.3020115420618266211, 0.1674077314120194226, -0.9384901064608612842 ) ) ;
#13039=ORIENTED_EDGE ( 'NONE', *, *, #12949, .T. ) ;
#13047=CARTESIAN_POINT ( 'NONE',  ( 70.12209330904275362, -3.652447179931426646, 75.96062414490636172 ) ) ;
#13048=CARTESIAN_POINT ( 'NONE',  ( 64.77204481361067678, -11.50071871444543881, 71.61353507035619259 ) ) ;
#13055=DIRECTION ( 'NONE',  ( -0.000000000000000000, 0.000000000000000000, -1.000000000000000000 ) ) ;
#13057=VERTEX_POINT ( 'NONE', #4374 ) ;
#13062=CARTESIAN_POINT ( 'NONE',  ( 66.24771997929842371, -11.54120404467442285, 76.19766410831375936 ) ) ;
#13066=ORIENTED_EDGE ( 'NONE', *, *, #8220, .T. ) ;
#13069=CIRCLE ( 'NONE', #4963, 7.924024642120691908 ) ;
#13072=TOROIDAL_SURFACE ( 'NONE', #15036, 2.000000000000000000, 1.000000000000000000 ) ;
#13074=CARTESIAN_POINT ( 'NONE',  ( 65.03656227622965957, -11.30130833895906406, 76.98918051064211454 ) ) ;
#13086=VECTOR ( 'NONE', #14240, 1000.000000000000000 ) ;
#13091=DIRECTION ( 'NONE',  ( 0.000000000000000000, 0.000000000000000000, 1.000000000000000000 ) ) ;
#13094=CIRCLE ( 'NONE', #8186, 11.46463184759105403 ) ;
#13098=VECTOR ( 'NONE', #8183, 1000.000000000000000 ) ;
#13103=VERTEX_POINT ( 'NONE', #7846 ) ;
#13112=DIRECTION ( 'NONE',  ( -0.8746197071345570562, 0.4848096202550665756, 0.000000000000000000 ) ) ;
#13122=CYLINDRICAL_SURFACE ( 'NONE', #5103, 0.7892041907098262810 ) ;
#13123=EDGE_CURVE ( 'NONE', #11609, #11588, #14557, .T. ) ;
#13125=CARTESIAN_POINT ( 'NONE',  ( 69.43199442225004248, -3.120433192335155592, 76.80468318204789568 ) ) ;
#13136=CARTESIAN_POINT ( 'NONE',  ( 65.13162939936435691, -11.91918766645189898, 75.26674478960599401 ) ) ;
#13140=EDGE_CURVE ( 'NONE', #5503, #7793, #2512, .T. ) ;
#13145=DIRECTION ( 'NONE',  ( -0.000000000000000000, 0.000000000000000000, -1.000000000000000000 ) ) ;
#13149=VERTEX_POINT ( 'NONE', #7768 ) ;
#13152=ORIENTED_EDGE ( 'NONE', *, *, #6390, .T. ) ;
#13154=ADVANCED_FACE ( 'NONE', ( #12454 ), #6757, .F. ) ;
#13159=DIRECTION ( 'NONE',  ( -0.000000000000000000, -0.000000000000000000, -1.000000000000000000 ) ) ;
#13168=CARTESIAN_POINT ( 'NONE',  ( 59.31076468612580754, 2.638779099491020297, 62.84860122826521689 ) ) ;
#13172=FACE_OUTER_BOUND ( 'NONE', #5307, .T. ) ;
#13178=EDGE_CURVE ( 'NONE', #7204, #8564, #6837, .T. ) ;
#13181=CARTESIAN_POINT ( 'NONE',  ( 56.56161818778031858, -7.613266777470379942, 60.61639468829817190 ) ) ;
#13194=CARTESIAN_POINT ( 'NONE',  ( 70.07305199753827196, -3.471083832564866967, 75.82119617954428747 ) ) ;
#13196=CIRCLE ( 'NONE', #2854, 1.000000000000001998 ) ;
#13216=ADVANCED_FACE ( 'NONE', ( #13008 ), #1136, .F. ) ;
#13222=ADVANCED_FACE ( 'NONE', ( #8383 ), #1775, .T. ) ;
#13229=VERTEX_POINT ( 'NONE', #3755 ) ;
#13233=ORIENTED_EDGE ( 'NONE', *, *, #8381, .T. ) ;
#13236=CIRCLE ( 'NONE', #14935, 8.924024642120691908 ) ;
#13245=CARTESIAN_POINT ( 'NONE',  ( 48.84742675818896629, 2.824063592853379046, 60.61639468829817190 ) ) ;
#13249=ORIENTED_EDGE ( 'NONE', *, *, #9895, .F. ) ;
#13255=CARTESIAN_POINT ( 'NONE',  ( 56.13062797998802722, -6.952138427283281352, 48.51982618741349285 ) ) ;
#13261=AXIS2_PLACEMENT_3D ( 'NONE', #8770, #14414, #12018 ) ;
#13264=ORIENTED_EDGE ( 'NONE', *, *, #14571, .T. ) ;
#13270=CARTESIAN_POINT ( 'NONE',  ( 70.04298944718500763, -3.369224104032832567, 75.71372953216713597 ) ) ;
#13274=ADVANCED_FACE ( 'NONE', ( #12930 ), #11984, .T. ) ;
#13275=CIRCLE ( 'NONE', #8594, 0.9999999999999954481 ) ;
#13290=CARTESIAN_POINT ( 'NONE',  ( 53.41380296247595538, -0.1096349785133995947, 60.61639468829817190 ) ) ;
#13297=ORIENTED_EDGE ( 'NONE', *, *, #11516, .T. ) ;
#13299=AXIS2_PLACEMENT_3D ( 'NONE', #8124, #4580, #2429 ) ;
#13300=EDGE_LOOP ( 'NONE', ( #7812, #9214, #5625, #8819 ) ) ;
#13307=VERTEX_POINT ( 'NONE', #6438 ) ;
#13309=CARTESIAN_POINT ( 'NONE',  ( 61.44362764059101067, -6.606194471396438672, 54.56811043785582882 ) ) ;
#13310=DIRECTION ( 'NONE',  ( -0.000000000000000000, 0.000000000000000000, -1.000000000000000000 ) ) ;
#13312=ORIENTED_EDGE ( 'NONE', *, *, #2868, .T. ) ;
#13325=DIRECTION ( 'NONE',  ( 0.000000000000000000, 0.000000000000000000, 1.000000000000000000 ) ) ;
#13328=CARTESIAN_POINT ( 'NONE',  ( 62.30678795759143185, -4.906903613034745426, 62.84860122826521689 ) ) ;
#13341=CARTESIAN_POINT ( 'NONE',  ( 65.71319926014255941, -10.73129157630437547, 71.19766410831374515 ) ) ;
#13345=EDGE_CURVE ( 'NONE', #4156, #3899, #2979, .T. ) ;
#13347=AXIS2_PLACEMENT_3D ( 'NONE', #10534, #12684, #2370 ) ;
#13349=EDGE_LOOP ( 'NONE', ( #12238, #10700 ) ) ;
#13352=ORIENTED_EDGE ( 'NONE', *, *, #10420, .T. ) ;
#13360=EDGE_CURVE ( 'NONE', #14177, #15000, #1530, .T. ) ;
#13368=ORIENTED_EDGE ( 'NONE', *, *, #11525, .F. ) ;
#13371=FACE_OUTER_BOUND ( 'NONE', #9624, .T. ) ;
#13374=CYLINDRICAL_SURFACE ( 'NONE', #10670, 0.7892041907098262810 ) ;
#13375=ORIENTED_EDGE ( 'NONE', *, *, #4991, .T. ) ;
#13378=CARTESIAN_POINT ( 'NONE',  ( 61.44362764059101067, -6.606194471396438672, 60.61639468829817190 ) ) ;
#13387=DIRECTION ( 'NONE',  ( 0.000000000000000000, 0.000000000000000000, 1.000000000000000000 ) ) ;
#13396=ADVANCED_FACE ( 'NONE', ( #1599 ), #9844, .T. ) ;
#13398=ORIENTED_EDGE ( 'NONE', *, *, #6195, .T. ) ;
#13401=AXIS2_PLACEMENT_3D ( 'NONE', #6554, #10030, #14790 ) ;
#13413=EDGE_LOOP ( 'NONE', ( #7101, #8481, #6311, #9789 ) ) ;
#13415=CYLINDRICAL_SURFACE ( 'NONE', #12583, 0.7892041907098262810 ) ;
#13424=VECTOR ( 'NONE', #3806, 1000.000000000000000 ) ;
#13428=ORIENTED_EDGE ( 'NONE', *, *, #8091, .F. ) ;
#13429=ORIENTED_EDGE ( 'NONE', *, *, #12088, .T. ) ;
#13433=ORIENTED_EDGE ( 'NONE', *, *, #7357, .F. ) ;
#13445=ORIENTED_EDGE ( 'NONE', *, *, #12360, .F. ) ;
#13452=CARTESIAN_POINT ( 'NONE',  ( 52.72354942432796321, 0.2729788054883383608, 62.84860122826521689 ) ) ;
#13455=VERTEX_POINT ( 'NONE', #6659 ) ;
#13459=AXIS2_PLACEMENT_3D ( 'NONE', #9014, #4475, #6705 ) ;
#13465=DIRECTION ( 'NONE',  ( 0.8746197071345569451, -0.4848096202550666312, 0.000000000000000000 ) ) ;
#13468=B_SPLINE_CURVE_WITH_KNOTS ( 'NONE', 3,
 ( #1229, #3616, #2466, #9631, #5866, #4848, #7155, #8164, #12867, #2313, #3543, #9556 ),
 .UNSPECIFIED., .F., .F.,
 ( 4, 2, 2, 2, 2, 4 ),
 ( 0.000000000000000000, 0.0002273805472697279430, 0.0004547610945394558860, 0.0009095221890789461413, 0.001364283283618436234, 0.001819044378157926543 ),
 .UNSPECIFIED. ) ;
#13473=CARTESIAN_POINT ( 'NONE',  ( 65.33616866150605063, -11.06260342404821628, 71.24779283330499879 ) ) ;
#13478=CARTESIAN_POINT ( 'NONE',  ( 56.97758043373130477, 2.707118148285912795, 48.51982618741349285 ) ) ;
#13486=EDGE_CURVE ( 'NONE', #8564, #996, #9378, .T. ) ;
#13489=AXIS2_PLACEMENT_3D ( 'NONE', #2711, #6474, #334 ) ;
#13494=ORIENTED_EDGE ( 'NONE', *, *, #15155, .T. ) ;
#13498=EDGE_LOOP ( 'NONE', ( #14820, #12068, #13375, #9786 ) ) ;
#13508=DIRECTION ( 'NONE',  ( 0.000000000000000000, 0.000000000000000000, 1.000000000000000000 ) ) ;
#13511=EDGE_LOOP ( 'NONE', ( #852, #8848, #3000, #11042 ) ) ;
#13518=CARTESIAN_POINT ( 'NONE',  ( 69.32502915396517551, -4.037540509912919795, 71.21138934095161233 ) ) ;
#13521=DIRECTION ( 'NONE',  ( 1.224646799147353207E-16, 1.000000000000000000, -0.000000000000000000 ) ) ;
#13525=VERTEX_POINT ( 'NONE', #11421 ) ;
#13526=FACE_OUTER_BOUND ( 'NONE', #11970, .T. ) ;
#13528=CYLINDRICAL_SURFACE ( 'NONE', #1314, 1.000000000000000888 ) ;
#13535=FACE_OUTER_BOUND ( 'NONE', #8687, .T. ) ;
#13540=AXIS2_PLACEMENT_3D ( 'NONE', #3493, #3332, #11644 ) ;
#13553=CIRCLE ( 'NONE', #12584, 11.46463184759105403 ) ;
#13557=DIRECTION ( 'NONE',  ( 0.000000000000000000, 0.000000000000000000, 1.000000000000000000 ) ) ;
#13559=DIRECTION ( 'NONE',  ( 0.8746197071345569451, -0.4848096202550666312, 0.000000000000000000 ) ) ;
#13562=AXIS2_PLACEMENT_3D ( 'NONE', #10944, #464, #2557 ) ;
#13566=DIRECTION ( 'NONE',  ( -1.000000000000000000, 0.000000000000000000, 0.000000000000000000 ) ) ;
#13575=ORIENTED_EDGE ( 'NONE', *, *, #3828, .T. ) ;
#13581=CARTESIAN_POINT ( 'NONE',  ( 56.97758043373130477, 2.707118148285912795, 62.84860122826521689 ) ) ;
#13586=CYLINDRICAL_SURFACE ( 'NONE', #199, 4.000000000000003553 ) ;
#13588=EDGE_LOOP ( 'NONE', ( #14919, #12732 ) ) ;
#13591=VERTEX_POINT ( 'NONE', #11897 ) ;
#13595=CARTESIAN_POINT ( 'NONE',  ( 69.46454297106447484, -2.294433322023681221, 73.06560708801610815 ) ) ;
#13599=DIRECTION ( 'NONE',  ( 0.8208219420614805140, -0.4549890321264307702, -0.3453061251629823691 ) ) ;
#13621=CARTESIAN_POINT ( 'NONE',  ( 66.24588231955848983, -11.54213538233861236, 72.19766410831374515 ) ) ;
#13633=LINE ( 'NONE', #775, #13954 ) ;
#13635=ORIENTED_EDGE ( 'NONE', *, *, #13123, .T. ) ;
#13649=EDGE_CURVE ( 'NONE', #7206, #7233, #11088, .T. ) ;
#13650=ORIENTED_EDGE ( 'NONE', *, *, #74, .T. ) ;
#13674=DIRECTION ( 'NONE',  ( 1.000000000000000000, 0.000000000000000000, 0.000000000000000000 ) ) ;
#13675=ORIENTED_EDGE ( 'NONE', *, *, #8381, .F. ) ;
#13687=VERTEX_POINT ( 'NONE', #12268 ) ;
#13690=EDGE_LOOP ( 'NONE', ( #4386, #13022, #12576, #12151 ) ) ;
#13699=DIRECTION ( 'NONE',  ( 0.8746197071345570562, -0.4848096202550665756, 0.000000000000000000 ) ) ;
#13706=CARTESIAN_POINT ( 'NONE',  ( 69.44125642334664406, -2.986918215369366081, 76.69762336658895663 ) ) ;
#13708=CARTESIAN_POINT ( 'NONE',  ( 57.83740799265796539, -7.800393779465814248, 54.56811043785582882 ) ) ;
#13710=ORIENTED_EDGE ( 'NONE', *, *, #10653, .F. ) ;
#13711=AXIS2_PLACEMENT_3D ( 'NONE', #11313, #2008, #11468 ) ;
#13712=CARTESIAN_POINT ( 'NONE',  ( 69.46051462023766021, -2.575682430178798832, 72.15988747666172287 ) ) ;
#13714=VERTEX_POINT ( 'NONE', #14368 ) ;
#13716=DIRECTION ( 'NONE',  ( 0.8746197071345569451, -0.4848096202550666312, 0.000000000000000000 ) ) ;
#13717=EDGE_LOOP ( 'NONE', ( #7375, #11118, #7062, #9255, #7317, #8960 ) ) ;
#13720=DIRECTION ( 'NONE',  ( 1.000000000000000000, 0.000000000000000000, 0.000000000000000000 ) ) ;
#13732=DIRECTION ( 'NONE',  ( -0.000000000000000000, 0.000000000000000000, -1.000000000000000000 ) ) ;
#13737=DIRECTION ( 'NONE',  ( 0.4848096202550658540, 0.8746197071345573892, 0.000000000000000000 ) ) ;
#13748=CIRCLE ( 'NONE', #7121, 0.7892041907098322762 ) ;
#13750=DIRECTION ( 'NONE',  ( 0.8746197071345560570, -0.4848096202550682410, 0.000000000000000000 ) ) ;
#13757=CARTESIAN_POINT ( 'NONE',  ( 66.11049071757111051, -11.60217708172952022, 76.17393377513106145 ) ) ;
#13759=CARTESIAN_POINT ( 'NONE',  ( 68.02719294894561131, -7.807454411681060691, 82.40005259842790508 ) ) ;
#13760=CARTESIAN_POINT ( 'NONE',  ( 59.12196317473677709, -7.688259372168277928, 60.61639468829817190 ) ) ;
#13761=ORIENTED_EDGE ( 'NONE', *, *, #4537, .F. ) ;
#13763=VERTEX_POINT ( 'NONE', #6215 ) ;
#13768=AXIS2_PLACEMENT_3D ( 'NONE', #12838, #11423, #13750 ) ;
#13775=DIRECTION ( 'NONE',  ( 0.000000000000000000, 0.000000000000000000, 1.000000000000000000 ) ) ;
#13780=CARTESIAN_POINT ( 'NONE',  ( 70.00558585377599741, -3.250648700864071206, 72.86275793890305863 ) ) ;
#13788=AXIS2_PLACEMENT_3D ( 'NONE', #3916, #5228, #9930 ) ;
#13789=DIRECTION ( 'NONE',  ( 0.000000000000000000, 0.000000000000000000, 1.000000000000000000 ) ) ;
#13790=CARTESIAN_POINT ( 'NONE',  ( 54.86190032082818391, 1.721056973166403603, 60.61639468829817190 ) ) ;
#13805=DIRECTION ( 'NONE',  ( -0.8746197071345569451, 0.4848096202550666312, 0.000000000000000000 ) ) ;
#13808=DIRECTION ( 'NONE',  ( 0.8746197071345560570, -0.4848096202550682410, 0.000000000000000000 ) ) ;
#13820=VECTOR ( 'NONE', #1072, 1000.000000000000000 ) ;
#13828=CARTESIAN_POINT ( 'NONE',  ( 70.26445833701072274, -4.474174595298148205, 76.19766410831374515 ) ) ;
#13842=ORIENTED_EDGE ( 'NONE', *, *, #2217, .T. ) ;
#13846=ORIENTED_EDGE ( 'NONE', *, *, #9195, .T. ) ;
#13848=VECTOR ( 'NONE', #12449, 1000.000000000000000 ) ;
#13853=CARTESIAN_POINT ( 'NONE',  ( 54.86190032082818391, 1.721056973166403603, 60.61639468829817190 ) ) ;
#13858=CARTESIAN_POINT ( 'NONE',  ( 54.03086304124234829, 0.8903401505190762233, 62.84860122826521689 ) ) ;
#13861=CARTESIAN_POINT ( 'NONE',  ( 69.43919918318417217, -3.018345010862574451, 71.67085758179622701 ) ) ;
#13864=LINE ( 'NONE', #13023, #4732 ) ;
#13868=DIRECTION ( 'NONE',  ( 0.8746197071345571672, -0.4848096202550660205, 0.000000000000000000 ) ) ;
#13873=EDGE_CURVE ( 'NONE', #6912, #3132, #6421, .T. ) ;
#13875=CARTESIAN_POINT ( 'NONE',  ( 52.35373241494735197, -0.8423457118892125894, 48.51982618741349285 ) ) ;
#13879=ORIENTED_EDGE ( 'NONE', *, *, #1881, .F. ) ;
#13887=DIRECTION ( 'NONE',  ( -0.8746197071345569451, 0.4848096202550666312, 0.000000000000000000 ) ) ;
#13893=CARTESIAN_POINT ( 'NONE',  ( 76.46532884418532205, -6.768019176512804158, 73.13615421477459222 ) ) ;
#13922=DIRECTION ( 'NONE',  ( -0.8746197071345572782, 0.4848096202550659650, 0.000000000000000000 ) ) ;
#13923=ORIENTED_EDGE ( 'NONE', *, *, #10733, .F. ) ;
#13928=VECTOR ( 'NONE', #796, 1000.000000000000000 ) ;
#13932=CARTESIAN_POINT ( 'NONE',  ( 65.13162939515778760, -11.91918766412016772, 73.05968396960713562 ) ) ;
#13938=FACE_OUTER_BOUND ( 'NONE', #12579, .T. ) ;
#13939=EDGE_CURVE ( 'NONE', #14247, #12141, #5947, .T. ) ;
#13941=AXIS2_PLACEMENT_3D ( 'NONE', #7190, #3573, #4734 ) ;
#13942=ORIENTED_EDGE ( 'NONE', *, *, #13939, .T. ) ;
#13953=VECTOR ( 'NONE', #2272, 999.9999999999998863 ) ;
#13954=VECTOR ( 'NONE', #5490, 1000.000000000000000 ) ;
#13969=CARTESIAN_POINT ( 'NONE',  ( 50.07597535787931520, -2.249290599286308368, 38.50000000000012790 ) ) ;
#13971=EDGE_CURVE ( 'NONE', #5118, #7249, #7883, .T. ) ;
#13992=DIRECTION ( 'NONE',  ( -0.000000000000000000, -0.000000000000000000, 1.000000000000000000 ) ) ;
#14008=VECTOR ( 'NONE', #1185, 1000.000000000000000 ) ;
#14016=ORIENTED_EDGE ( 'NONE', *, *, #4382, .F. ) ;
#14017=CARTESIAN_POINT ( 'NONE',  ( 75.52271037289314393, -7.388871293676331220, 72.19766410831374515 ) ) ;
#14019=ORIENTED_EDGE ( 'NONE', *, *, #10223, .T. ) ;
#14024=ORIENTED_EDGE ( 'NONE', *, *, #9971, .F. ) ;
#14035=EDGE_CURVE ( 'NONE', #11155, #5118, #14056, .T. ) ;
#14036=EDGE_LOOP ( 'NONE', ( #8742, #6603, #12368, #4428 ) ) ;
#14045=AXIS2_PLACEMENT_3D ( 'NONE', #10576, #8193, #4723 ) ;
#14046=CIRCLE ( 'NONE', #1005, 0.7892041907098286124 ) ;
#14050=B_SPLINE_CURVE_WITH_KNOTS ( 'NONE', 3,
 ( #742, #14904, #10376, #4365, #4523, #5452, #10146, #7837, #15075, #13757, #14834, #10300 ),
 .UNSPECIFIED., .F., .F.,
 ( 4, 2, 2, 2, 2, 4 ),
 ( 0.000000000000000000, 0.0002273805472697271570, 0.0004547610945394543139, 0.0009095221890789429971, 0.001364283283618431463, 0.001819044378157920255 ),
 .UNSPECIFIED. ) ;
#14056=CIRCLE ( 'NONE', #3724, 0.9999999999999963363 ) ;
#14057=VECTOR ( 'NONE', #6165, 1000.000000000000000 ) ;
#14064=LINE ( 'NONE', #7208, #5216 ) ;
#14069=VERTEX_POINT ( 'NONE', #4881 ) ;
#14081=DIRECTION ( 'NONE',  ( 0.4848096202550659650, 0.8746197071345572782, -0.000000000000000000 ) ) ;
#14082=VERTEX_POINT ( 'NONE', #15194 ) ;
#14088=CARTESIAN_POINT ( 'NONE',  ( 68.02719294894561131, -7.807454411681060691, 61.61639468829817190 ) ) ;
#14090=EDGE_LOOP ( 'NONE', ( #10343, #225, #8812, #4488 ) ) ;
#14098=CARTESIAN_POINT ( 'NONE',  ( 70.18619815789806182, -3.934114537491368857, 72.29468792547720568 ) ) ;
#14099=AXIS2_PLACEMENT_3D ( 'NONE', #14246, #7236, #4930 ) ;
#14102=FACE_OUTER_BOUND ( 'NONE', #2321, .T. ) ;
#14105=CARTESIAN_POINT ( 'NONE',  ( 62.14609464170151654, 0.6526447315840442354, 62.84860122826521689 ) ) ;
#14107=ORIENTED_EDGE ( 'NONE', *, *, #8044, .T. ) ;
#14111=DIRECTION ( 'NONE',  ( -0.000000000000000000, 0.000000000000000000, -1.000000000000000000 ) ) ;
#14120=CARTESIAN_POINT ( 'NONE',  ( 118.2606911748681568, -35.65233716510192608, 53.46824312087640863 ) ) ;
#14121=VERTEX_POINT ( 'NONE', #7336 ) ;
#14122=EDGE_CURVE ( 'NONE', #943, #11350, #2574, .T. ) ;
#14124=CARTESIAN_POINT ( 'NONE',  ( 53.45023817967523172, -5.433760736713491468, 54.56811043785582882 ) ) ;
#14142=CARTESIAN_POINT ( 'NONE',  ( 65.33089625181217741, -11.07072041448327226, 76.23223904883872137 ) ) ;
#14151=ORIENTED_EDGE ( 'NONE', *, *, #6409, .T. ) ;
#14152=CARTESIAN_POINT ( 'NONE',  ( 64.20382552624532480, -11.89050466264470529, 75.84179418424443497 ) ) ;
#14175=DIRECTION ( 'NONE',  ( 0.000000000000000000, 0.000000000000000000, 1.000000000000000000 ) ) ;
#14177=VERTEX_POINT ( 'NONE', #2643 ) ;
#14185=DIRECTION ( 'NONE',  ( -1.387778780781444413E-14, 1.127570259384923665E-14, -1.000000000000000000 ) ) ;
#14188=CYLINDRICAL_SURFACE ( 'NONE', #7362, 0.7892041907098261699 ) ;
#14193=ORIENTED_EDGE ( 'NONE', *, *, #11099, .F. ) ;
#14195=CARTESIAN_POINT ( 'NONE',  ( 58.00000000000000711, -2.249290599286309256, 61.61639468829817190 ) ) ;
#14198=CARTESIAN_POINT ( 'NONE',  ( 56.25419740419757630, 3.022649838004307199, 54.56811043785582882 ) ) ;
#14200=MANIFOLD_SOLID_BREP ( 'Boss-Extrude16', #8786 ) ;
#14204=AXIS2_PLACEMENT_3D ( 'NONE', #3940, #1787, #13559 ) ;
#14206=CARTESIAN_POINT ( 'NONE',  ( 64.46753801043549004, -11.71576859601145593, 71.98115573486096253 ) ) ;
#14218=CARTESIAN_POINT ( 'NONE',  ( 65.51024544200237187, -10.91545772570538553, 76.25780573704503240 ) ) ;
#14219=DIRECTION ( 'NONE',  ( 0.000000000000000000, 0.000000000000000000, 1.000000000000000000 ) ) ;
#14220=CARTESIAN_POINT ( 'NONE',  ( 61.18622467607353599, 2.299242679852278481, 60.61639468829817190 ) ) ;
#14221=AXIS2_PLACEMENT_3D ( 'NONE', #12702, #10472, #12872 ) ;
#14230=ORIENTED_EDGE ( 'NONE', *, *, #6742, .F. ) ;
#14231=CARTESIAN_POINT ( 'NONE',  ( 56.13062797998802722, -6.952138427283281352, 62.84860122826521689 ) ) ;
#14237=DIRECTION ( 'NONE',  ( -0.8746197071345572782, 0.4848096202550659650, 0.000000000000000000 ) ) ;
#14240=DIRECTION ( 'NONE',  ( 0.4848096202550659650, 0.8746197071345572782, -0.000000000000000000 ) ) ;
#14246=CARTESIAN_POINT ( 'NONE',  ( 54.03086304124234829, 0.8903401505190762233, 48.51982618741349285 ) ) ;
#14247=VERTEX_POINT ( 'NONE', #6777 ) ;
#14250=EDGE_LOOP ( 'NONE', ( #6437, #1023, #1617, #317 ) ) ;
#14254=AXIS2_PLACEMENT_3D ( 'NONE', #6412, #9961, #13566 ) ;
#14258=DIRECTION ( 'NONE',  ( 0.8208219420614746298, -0.4549890321264247195, -0.3453061251630045736 ) ) ;
#14263=DIRECTION ( 'NONE',  ( 0.3020115420618164626, -0.1674077314120084592, 0.9384901064608666132 ) ) ;
#14273=FACE_OUTER_BOUND ( 'NONE', #9621, .T. ) ;
#14283=CARTESIAN_POINT ( 'NONE',  ( 60.05137561479872232, 2.911430354694811484, 54.56811043785582882 ) ) ;
#14286=VERTEX_POINT ( 'NONE', #695 ) ;
#14288=CARTESIAN_POINT ( 'NONE',  ( 58.00000000000000711, -2.249290599286309256, 86.40005259842790508 ) ) ;
#14289=CARTESIAN_POINT ( 'NONE',  ( 58.00000000000000711, -2.249290599286309256, 39.50000000000012790 ) ) ;
#14303=ORIENTED_EDGE ( 'NONE', *, *, #9520, .T. ) ;
#14319=ORIENTED_EDGE ( 'NONE', *, *, #4323, .F. ) ;
#14320=EDGE_CURVE ( 'NONE', #12939, #6522, #10479, .T. ) ;
#14328=CIRCLE ( 'NONE', #2526, 0.7892041907098262810 ) ;
#14332=CARTESIAN_POINT ( 'NONE',  ( 54.86190032082818391, 1.721056973166403603, 48.51982618741349285 ) ) ;
#14334=ADVANCED_FACE ( 'NONE', ( #4472 ), #3631, .T. ) ;
#14345=DIRECTION ( 'NONE',  ( -1.000000000000000000, 0.000000000000000000, 0.000000000000000000 ) ) ;
#14353=ADVANCED_FACE ( 'NONE', ( #8178 ), #15043, .T. ) ;
#14356=FACE_OUTER_BOUND ( 'NONE', #7474, .T. ) ;
#14358=CARTESIAN_POINT ( 'NONE',  ( 69.32560489365786793, -4.047139788659277926, 77.19766409531744955 ) ) ;
#14367=ORIENTED_EDGE ( 'NONE', *, *, #207, .T. ) ;
#14368=CARTESIAN_POINT ( 'NONE',  ( 52.46774229227035136, -1.764205727211077379, 60.61639468829817190 ) ) ;
#14369=ORIENTED_EDGE ( 'NONE', *, *, #8145, .F. ) ;
#14371=CARTESIAN_POINT ( 'NONE',  ( 65.21119105374334879, -11.89996587754543711, 75.53257027772512799 ) ) ;
#14373=EDGE_CURVE ( 'NONE', #14748, #3495, #13864, .T. ) ;
#14382=DIRECTION ( 'NONE',  ( -1.000000000000000000, 0.000000000000000000, 0.000000000000000000 ) ) ;
#14393=DIRECTION ( 'NONE',  ( 0.000000000000000000, 0.000000000000000000, 1.000000000000000000 ) ) ;
#14404=ADVANCED_FACE ( 'NONE', ( #12880 ), #7168, .T. ) ;
#14409=DIRECTION ( 'NONE',  ( 0.4848096202550659650, 0.8746197071345572782, -0.000000000000000000 ) ) ;
#14414=DIRECTION ( 'NONE',  ( -0.4848096202550659650, -0.8746197071345572782, 0.000000000000000000 ) ) ;
#14435=UNCERTAINTY_MEASURE_WITH_UNIT (LENGTH_MEASURE( 1.000000000000000082E-05 ), #2945, 'distance_accuracy_value', 'NONE');
#14444=CYLINDRICAL_SURFACE ( 'NONE', #1147, 8.924024642120684803 ) ;
#14450=AXIS2_PLACEMENT_3D ( 'NONE', #15104, #13789, #3247 ) ;
#14454=VERTEX_POINT ( 'NONE', #248 ) ;
#14470=PLANE ( 'NONE',  #13788 ) ;
#14474=CARTESIAN_POINT ( 'NONE',  ( 66.38598137497019991, -11.47113225237460910, 72.19766410831374515 ) ) ;
#14495=DIRECTION ( 'NONE',  ( 0.8746197071345572782, -0.4848096202550659650, 0.000000000000000000 ) ) ;
#14496=EDGE_CURVE ( 'NONE', #4156, #10163, #7430, .T. ) ;
#14497=EDGE_CURVE ( 'NONE', #13455, #3217, #9865, .T. ) ;
#14498=PLANE ( 'NONE',  #3593 ) ;
#14500=CARTESIAN_POINT ( 'NONE',  ( 64.17080745393407426, -11.91156998299096337, 72.67649750183591095 ) ) ;
#14502=EDGE_CURVE ( 'NONE', #6181, #1998, #13094, .T. ) ;
#14504=ORIENTED_EDGE ( 'NONE', *, *, #9296, .F. ) ;
#14511=CARTESIAN_POINT ( 'NONE',  ( 58.00000000000000711, -2.249290599286309256, 47.51982618741348574 ) ) ;
#14523=CARTESIAN_POINT ( 'NONE',  ( 62.70356846721307420, -0.3817325368051065482, 62.84860122826521689 ) ) ;
#14536=AXIS2_PLACEMENT_3D ( 'NONE', #11262, #7816, #13808 ) ;
#14549=DIRECTION ( 'NONE',  ( 0.000000000000000000, 0.000000000000000000, 1.000000000000000000 ) ) ;
#14553=EDGE_CURVE ( 'NONE', #10521, #3380, #10386, .T. ) ;
#14556=CARTESIAN_POINT ( 'NONE',  ( 57.26556849154462725, -7.256479411572841265, 48.51982618741349285 ) ) ;
#14557=CIRCLE ( 'NONE', #5220, 1.000000000000007550 ) ;
#14570=CIRCLE ( 'NONE', #5736, 1.000000000000001554 ) ;
#14571=EDGE_CURVE ( 'NONE', #612, #6145, #15054, .T. ) ;
#14578=ORIENTED_EDGE ( 'NONE', *, *, #1040, .T. ) ;
#14580=EDGE_LOOP ( 'NONE', ( #2990, #8148, #12910, #761 ) ) ;
#14583=EDGE_CURVE ( 'NONE', #11220, #14995, #8841, .T. ) ;
#14586=AXIS2_PLACEMENT_3D ( 'NONE', #152, #10545, #14237 ) ;
#14587=DIRECTION ( 'NONE',  ( 0.8746197071345572782, -0.4848096202550659650, 0.000000000000000000 ) ) ;
#14589=ADVANCED_FACE ( 'NONE', ( #13535 ), #14613, .T. ) ;
#14595=ORIENTED_EDGE ( 'NONE', *, *, #13486, .F. ) ;
#14597=CARTESIAN_POINT ( 'NONE',  ( 69.40535631463106370, -3.419795260923345293, 71.40614770598537575 ) ) ;
#14604=DIRECTION ( 'NONE',  ( -0.000000000000000000, 0.000000000000000000, -1.000000000000000000 ) ) ;
#14607=VERTEX_POINT ( 'NONE', #1051 ) ;
#14613=SPHERICAL_SURFACE ( 'NONE', #5730, 1.000000000000000000 ) ;
#14620=CARTESIAN_POINT ( 'NONE',  ( 65.32988938321494743, -11.07158469721469629, 72.16329424003777149 ) ) ;
#14633=CARTESIAN_POINT ( 'NONE',  ( 58.00000000000000711, -2.249290599286309256, 71.19766410831374515 ) ) ;
#14636=DIRECTION ( 'NONE',  ( 0.000000000000000000, 0.000000000000000000, 1.000000000000000000 ) ) ;
#14640=CIRCLE ( 'NONE', #3345, 0.7892041907098262810 ) ;
#14641=ORIENTED_EDGE ( 'NONE', *, *, #8145, .T. ) ;
#14646=FACE_OUTER_BOUND ( 'NONE', #506, .T. ) ;
#14654=CYLINDRICAL_SURFACE ( 'NONE', #2243, 0.7892041907098262810 ) ;
#14661=ORIENTED_EDGE ( 'NONE', *, *, #10450, .F. ) ;
#14662=CIRCLE ( 'NONE', #2133, 0.7892041907098263920 ) ;
#14666=ORIENTED_EDGE ( 'NONE', *, *, #706, .F. ) ;
#14668=CARTESIAN_POINT ( 'NONE',  ( 69.46098093241307936, -2.556544511925992857, 72.19317000922296756 ) ) ;
#14669=AXIS2_PLACEMENT_3D ( 'NONE', #7920, #5535, #10220 ) ;
#14675=EDGE_CURVE ( 'NONE', #10980, #11609, #14064, .T. ) ;
#14681=DIRECTION ( 'NONE',  ( 0.000000000000000000, 0.000000000000000000, -1.000000000000000000 ) ) ;
#14686=ORIENTED_EDGE ( 'NONE', *, *, #4364, .T. ) ;
#14687=PRODUCT_DEFINITION_SHAPE ( 'NONE', 'NONE',  #5056 ) ;
#14688=CIRCLE ( 'NONE', #1425, 0.7892041907098262810 ) ;
#14692=DIRECTION ( 'NONE',  ( 0.8746197071345572782, -0.4848096202550659650, 0.000000000000000000 ) ) ;
#14700=CARTESIAN_POINT ( 'NONE',  ( 60.05137561479872232, 2.911430354694811484, 60.61639468829817190 ) ) ;
#14702=EDGE_CURVE ( 'NONE', #12099, #3816, #3977, .T. ) ;
#14711=DIRECTION ( 'NONE',  ( 0.000000000000000000, 0.000000000000000000, 1.000000000000000000 ) ) ;
#14715=ADVANCED_FACE ( 'NONE', ( #1118 ), #9915, .F. ) ;
#14718=AXIS2_PLACEMENT_3D ( 'NONE', #2093, #7724, #12409 ) ;
#14719=AXIS2_PLACEMENT_3D ( 'NONE', #7799, #12492, #11321 ) ;
#14726=ORIENTED_EDGE ( 'NONE', *, *, #5966, .T. ) ;
#14737=CIRCLE ( 'NONE', #9611, 5.496540510819668768 ) ;
#14740=ORIENTED_EDGE ( 'NONE', *, *, #12360, .T. ) ;
#14746=DIRECTION ( 'NONE',  ( -0.000000000000000000, 0.000000000000000000, -1.000000000000000000 ) ) ;
#14748=VERTEX_POINT ( 'NONE', #10973 ) ;
#14749=AXIS2_PLACEMENT_3D ( 'NONE', #14794, #12262, #5266 ) ;
#14751=ORIENTED_EDGE ( 'NONE', *, *, #12529, .T. ) ;
#14755=FACE_OUTER_BOUND ( 'NONE', #4040, .T. ) ;
#14763=CARTESIAN_POINT ( 'NONE',  ( 76.14589960879430919, -7.734310727912411920, 75.19766410831374515 ) ) ;
#14774=CARTESIAN_POINT ( 'NONE',  ( 64.48765185601422445, -11.70201852112108121, 71.95059996449334960 ) ) ;
#14780=VECTOR ( 'NONE', #12111, 1000.000000000000000 ) ;
#14781=CARTESIAN_POINT ( 'NONE',  ( 63.43853564383336874, -3.373351419973840581, 60.61639468829817190 ) ) ;
#14790=DIRECTION ( 'NONE',  ( 0.000000000000000000, 0.000000000000000000, -1.000000000000000000 ) ) ;
#14794=CARTESIAN_POINT ( 'NONE',  ( 56.13062797998802722, -6.952138427283281352, 60.61639468829817190 ) ) ;
#14820=ORIENTED_EDGE ( 'NONE', *, *, #9001, .F. ) ;
#14824=EDGE_CURVE ( 'NONE', #3324, #6435, #11608, .T. ) ;
#14834=CARTESIAN_POINT ( 'NONE',  ( 66.24913411760721260, -11.54048735118959002, 76.19766410831375936 ) ) ;
#14840=VERTEX_POINT ( 'NONE', #9828 ) ;
#14841=DIRECTION ( 'NONE',  ( -0.8208219420614786266, 0.4549890321264269399, 0.3453061251629920281 ) ) ;
#14849=FACE_OUTER_BOUND ( 'NONE', #518, .T. ) ;
#14854=CARTESIAN_POINT ( 'NONE',  ( 69.99597282625204286, -3.221539741904409837, 72.92829229118105161 ) ) ;
#14855=EDGE_CURVE ( 'NONE', #8583, #14121, #1659, .T. ) ;
#14867=EDGE_CURVE ( 'NONE', #9708, #13714, #8903, .T. ) ;
#14878=VERTEX_POINT ( 'NONE', #947 ) ;
#14879=DIRECTION ( 'NONE',  ( 0.8746197071345569451, -0.4848096202550666312, 0.000000000000000000 ) ) ;
#14904=CARTESIAN_POINT ( 'NONE',  ( 65.13162939602318602, -11.91918766459985157, 75.27488260206156667 ) ) ;
#14909=ORIENTED_EDGE ( 'NONE', *, *, #5178, .F. ) ;
#14915=AXIS2_PLACEMENT_3D ( 'NONE', #9667, #5174, #12027 ) ;
#14918=AXIS2_PLACEMENT_3D ( 'NONE', #11452, #10087, #5627 ) ;
#14919=ORIENTED_EDGE ( 'NONE', *, *, #1119, .T. ) ;
#14921=DIRECTION ( 'NONE',  ( -0.4848096202550659650, -0.8746197071345572782, 0.000000000000000000 ) ) ;
#14930=CARTESIAN_POINT ( 'NONE',  ( 76.00751999314820750, -6.514251586541772276, 73.19766410831374515 ) ) ;
#14931=CARTESIAN_POINT ( 'NONE',  ( 69.37814714961265850, -3.660029812082665313, 77.09164763542320031 ) ) ;
#14933=DIRECTION ( 'NONE',  ( -0.000000000000000000, 0.000000000000000000, -1.000000000000000000 ) ) ;
#14935=AXIS2_PLACEMENT_3D ( 'NONE', #15031, #9189, #13720 ) ;
#14947=DIRECTION ( 'NONE',  ( -0.000000000000000000, -0.000000000000000000, -1.000000000000000000 ) ) ;
#14952=CYLINDRICAL_SURFACE ( 'NONE', #4626, 0.7892041907098262810 ) ;
#14969=EDGE_CURVE ( 'NONE', #9315, #5234, #5983, .T. ) ;
#14974=CARTESIAN_POINT ( 'NONE',  ( 58.00000000000000711, -2.249290599286309256, 39.50000000000012790 ) ) ;
#14977=ORIENTED_EDGE ( 'NONE', *, *, #9628, .T. ) ;
#14987=ADVANCED_FACE ( 'NONE', ( #11569 ), #3185, .T. ) ;
#14988=DIRECTION ( 'NONE',  ( -0.000000000000000000, -0.000000000000000000, -1.000000000000000000 ) ) ;
#14995=VERTEX_POINT ( 'NONE', #4497 ) ;
#14998=ORIENTED_EDGE ( 'NONE', *, *, #13486, .T. ) ;
#15000=VERTEX_POINT ( 'NONE', #12581 ) ;
#15008=DIRECTION ( 'NONE',  ( 0.000000000000000000, 0.000000000000000000, 1.000000000000000000 ) ) ;
#15009=ORIENTED_EDGE ( 'NONE', *, *, #5025, .T. ) ;
#15014=CARTESIAN_POINT ( 'NONE',  ( 52.72873328492558187, -0.5014548242779810483, 60.61639468829817190 ) ) ;
#15017=CARTESIAN_POINT ( 'NONE',  ( 70.22813770118101218, -4.160309161658024557, 72.22283181065139956 ) ) ;
#15023=ADVANCED_FACE ( 'NONE', ( #14273 ), #15122, .T. ) ;
#15030=AXIS2_PLACEMENT_3D ( 'NONE', #711, #7806, #5505 ) ;
#15031=CARTESIAN_POINT ( 'NONE',  ( 58.00000000000000711, -2.249290599286309256, 39.50000000000012790 ) ) ;
#15036=AXIS2_PLACEMENT_3D ( 'NONE', #12977, #11732, #4654 ) ;
#15039=ORIENTED_EDGE ( 'NONE', *, *, #7164, .F. ) ;
#15043=TOROIDAL_SURFACE ( 'NONE', #1534, 7.924024642120688355, 1.000000000000000000 ) ;
#15044=DIRECTION ( 'NONE',  ( 0.000000000000000000, 0.000000000000000000, 1.000000000000000000 ) ) ;
#15050=DIRECTION ( 'NONE',  ( -0.8746197071345570562, 0.4848096202550665756, 0.000000000000000000 ) ) ;
#15053=CARTESIAN_POINT ( 'NONE',  ( 62.35557539207178479, -5.694598376804811402, 60.61639468829817190 ) ) ;
#15054=CIRCLE ( 'NONE', #1546, 10.46463184759104692 ) ;
#15075=CARTESIAN_POINT ( 'NONE',  ( 65.83900612928935914, -11.71016173102437818, 76.08636588808168710 ) ) ;
#15082=DIRECTION ( 'NONE',  ( -0.3020115420618249003, 0.1674077314120184790, -0.9384901064608620613 ) ) ;
#15089=DIRECTION ( 'NONE',  ( -0.000000000000000000, -0.000000000000000000, 1.000000000000000000 ) ) ;
#15098=CARTESIAN_POINT ( 'NONE',  ( 69.39833270110392505, -3.557321787083441489, 72.23228168306333430 ) ) ;
#15102=ORIENTED_EDGE ( 'NONE', *, *, #11525, .T. ) ;
#15104=CARTESIAN_POINT ( 'NONE',  ( 58.00000000000000711, -2.249290599286309256, 72.19766410831374515 ) ) ;
#15107=ORIENTED_EDGE ( 'NONE', *, *, #14122, .F. ) ;
#15113=CARTESIAN_POINT ( 'NONE',  ( 121.5907739023289622, -31.78146182366518957, 56.28371344025897827 ) ) ;
#15118=ORIENTED_EDGE ( 'NONE', *, *, #3409, .F. ) ;
#15122=CYLINDRICAL_SURFACE ( 'NONE', #553, 0.7892041907098262810 ) ;
#15126=CARTESIAN_POINT ( 'NONE',  ( 52.50499674461036648, -3.053107681157296582, 54.56811043785582882 ) ) ;
#15128=CYLINDRICAL_SURFACE ( 'NONE', #13299, 1.000000000000000888 ) ;
#15136=ORIENTED_EDGE ( 'NONE', *, *, #12236, .F. ) ;
#15141=ORIENTED_EDGE ( 'NONE', *, *, #10897, .F. ) ;
#15143=DIRECTION ( 'NONE',  ( 0.000000000000000000, 0.000000000000000000, 1.000000000000000000 ) ) ;
#15145=DIRECTION ( 'NONE',  ( 0.8746197071345569451, -0.4848096202550666312, 0.000000000000000000 ) ) ;
#15150=ORIENTED_EDGE ( 'NONE', *, *, #10509, .F. ) ;
#15154=EDGE_CURVE ( 'NONE', #5063, #13149, #6553, .T. ) ;
#15155=EDGE_CURVE ( 'NONE', #11686, #14069, #5896, .T. ) ;
#15157=LINE ( 'NONE', #10772, #5508 ) ;
#15165=CARTESIAN_POINT ( 'NONE',  ( 62.70356846721307420, -0.3817325368051065482, 48.51982618741349285 ) ) ;
#15167=DIRECTION ( 'NONE',  ( 0.8208219420614786266, -0.4549890321264268289, -0.3453061251629919726 ) ) ;
#15171=EDGE_CURVE ( 'NONE', #3763, #2576, #11801, .T. ) ;
#15172=CIRCLE ( 'NONE', #1884, 8.924024642120691908 ) ;
#15174=DIRECTION ( 'NONE',  ( 0.3020115420618249003, -0.1674077314120184790, 0.9384901064608621724 ) ) ;
#15177=DIRECTION ( 'NONE',  ( -0.000000000000000000, -0.000000000000000000, 1.000000000000000000 ) ) ;
#15179=ORIENTED_EDGE ( 'NONE', *, *, #14675, .T. ) ;
#15188=CARTESIAN_POINT ( 'NONE',  ( 61.36510378087922390, 1.530577915148011225, 62.84860122826521689 ) ) ;
#15192=DIRECTION ( 'NONE',  ( 0.000000000000000000, 0.000000000000000000, 1.000000000000000000 ) ) ;
#15194=CARTESIAN_POINT ( 'NONE',  ( 56.25419740419757630, 3.022649838004307199, 48.51982618741349285 ) ) ;
#15202=CARTESIAN_POINT ( 'NONE',  ( 53.04398595309534414, -1.224959495890951100, 62.84860122826521689 ) ) ;
#15217=EDGE_CURVE ( 'NONE', #15000, #59, #4086, .T. ) ;
#15223=DIRECTION ( 'NONE',  ( 0.000000000000000000, 0.000000000000000000, 1.000000000000000000 ) ) ;
#15273=COLOUR_RGB('Off White',0.89,0.88,0.83);
#15274=FILL_AREA_STYLE_COLOUR('',#15273);
#15275=FILL_AREA_STYLE('',(#15274));
#15276=SURFACE_STYLE_FILL_AREA(#15275);
#15277=SURFACE_SIDE_STYLE('',(#15276));
#15278=SURFACE_STYLE_USAGE(.BOTH.,#15277);
#15279=PRESENTATION_STYLE_ASSIGNMENT((#15278));
ENDSEC;
END-ISO-10303-21;
